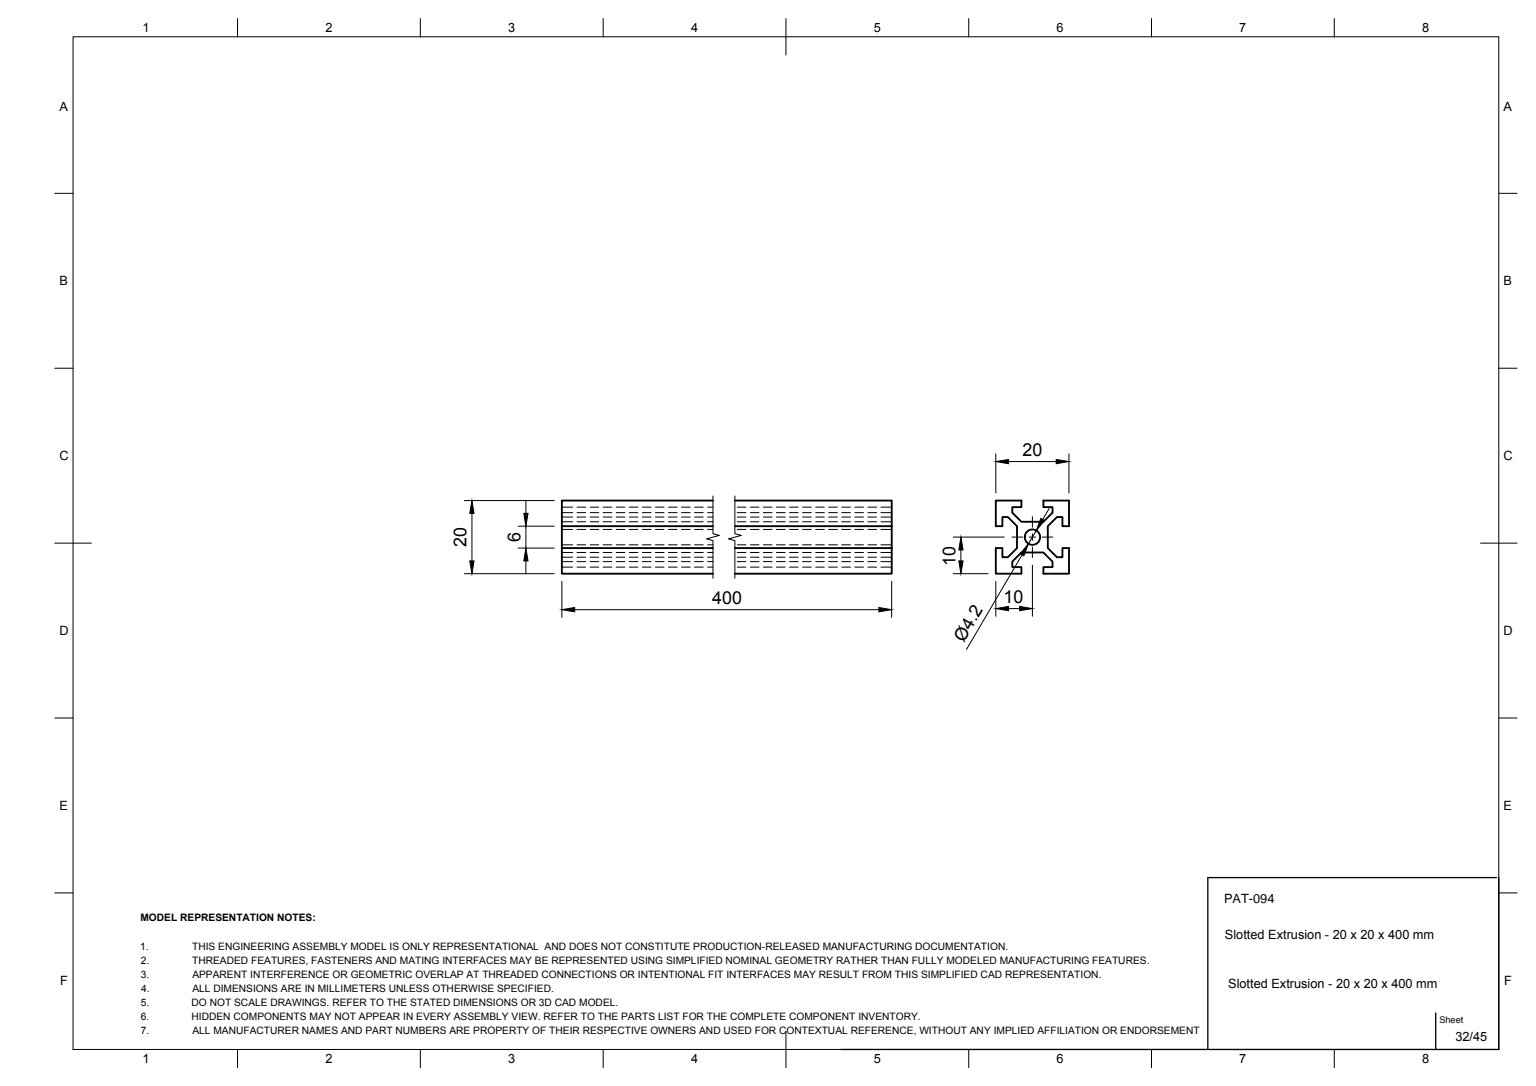
ISO-10303-21;
HEADER;
/* Generated by software containing ST-Developer
 * from STEP Tools, Inc. (www.steptools.com) 
 */

FILE_DESCRIPTION(
/* description */ ('Shaft runout checking stand'),
/* implementation_level */ '2;1');

FILE_NAME(
/* name */ 'Slotted Extrusion - 20 x 20 x 400 mm.step',
/* time_stamp */ '2026-11-02T21:12:33-08:00',
/* author */ (''),
/* organization */ (''),
/* preprocessor_version */ 'ST-DEVELOPER v20.2',
/* originating_system */ 'Autodesk Translation Framework v15.17.0.0',
/* authorisation */ '');

FILE_SCHEMA (('AUTOMOTIVE_DESIGN { 1 0 10303 214 3 1 1 }'));
ENDSEC;

DATA;
#10=MECHANICAL_DESIGN_GEOMETRIC_PRESENTATION_REPRESENTATION('',(#463),#11748);
#377=SHAPE_REPRESENTATION_RELATIONSHIP('SRR','None',#11926,#420);
#420=ADVANCED_BREP_SHAPE_REPRESENTATION('',(#514),#11702);
#463=STYLED_ITEM('',(#12169),#514);
#514=MANIFOLD_SOLID_BREP('Body1',#6206);
#562=FACE_BOUND('',#1452,.T.);
#563=FACE_BOUND('',#1454,.T.);
#673=CIRCLE('',#6774,0.21);
#674=CIRCLE('',#6775,0.21);
#938=CYLINDRICAL_SURFACE('',#6773,0.21);
#1038=FACE_OUTER_BOUND('',#1406,.T.);
#1039=FACE_OUTER_BOUND('',#1407,.T.);
#1040=FACE_OUTER_BOUND('',#1408,.T.);
#1041=FACE_OUTER_BOUND('',#1409,.T.);
#1042=FACE_OUTER_BOUND('',#1410,.T.);
#1043=FACE_OUTER_BOUND('',#1411,.T.);
#1044=FACE_OUTER_BOUND('',#1412,.T.);
#1045=FACE_OUTER_BOUND('',#1413,.T.);
#1046=FACE_OUTER_BOUND('',#1414,.T.);
#1047=FACE_OUTER_BOUND('',#1415,.T.);
#1048=FACE_OUTER_BOUND('',#1416,.T.);
#1049=FACE_OUTER_BOUND('',#1417,.T.);
#1050=FACE_OUTER_BOUND('',#1418,.T.);
#1051=FACE_OUTER_BOUND('',#1419,.T.);
#1052=FACE_OUTER_BOUND('',#1420,.T.);
#1053=FACE_OUTER_BOUND('',#1421,.T.);
#1054=FACE_OUTER_BOUND('',#1422,.T.);
#1055=FACE_OUTER_BOUND('',#1423,.T.);
#1056=FACE_OUTER_BOUND('',#1424,.T.);
#1057=FACE_OUTER_BOUND('',#1425,.T.);
#1058=FACE_OUTER_BOUND('',#1426,.T.);
#1059=FACE_OUTER_BOUND('',#1427,.T.);
#1060=FACE_OUTER_BOUND('',#1428,.T.);
#1061=FACE_OUTER_BOUND('',#1429,.T.);
#1062=FACE_OUTER_BOUND('',#1430,.T.);
#1063=FACE_OUTER_BOUND('',#1431,.T.);
#1064=FACE_OUTER_BOUND('',#1432,.T.);
#1065=FACE_OUTER_BOUND('',#1433,.T.);
#1066=FACE_OUTER_BOUND('',#1434,.T.);
#1067=FACE_OUTER_BOUND('',#1435,.T.);
#1068=FACE_OUTER_BOUND('',#1436,.T.);
#1069=FACE_OUTER_BOUND('',#1437,.T.);
#1070=FACE_OUTER_BOUND('',#1438,.T.);
#1071=FACE_OUTER_BOUND('',#1439,.T.);
#1072=FACE_OUTER_BOUND('',#1440,.T.);
#1073=FACE_OUTER_BOUND('',#1441,.T.);
#1074=FACE_OUTER_BOUND('',#1442,.T.);
#1075=FACE_OUTER_BOUND('',#1443,.T.);
#1076=FACE_OUTER_BOUND('',#1444,.T.);
#1077=FACE_OUTER_BOUND('',#1445,.T.);
#1078=FACE_OUTER_BOUND('',#1446,.T.);
#1079=FACE_OUTER_BOUND('',#1447,.T.);
#1080=FACE_OUTER_BOUND('',#1448,.T.);
#1081=FACE_OUTER_BOUND('',#1449,.T.);
#1082=FACE_OUTER_BOUND('',#1450,.T.);
#1083=FACE_OUTER_BOUND('',#1451,.T.);
#1084=FACE_OUTER_BOUND('',#1453,.T.);
#1406=EDGE_LOOP('',(#4088,#4089,#4090,#4091));
#1407=EDGE_LOOP('',(#4092,#4093,#4094,#4095));
#1408=EDGE_LOOP('',(#4096,#4097,#4098,#4099));
#1409=EDGE_LOOP('',(#4100,#4101,#4102,#4103));
#1410=EDGE_LOOP('',(#4104,#4105,#4106,#4107));
#1411=EDGE_LOOP('',(#4108,#4109,#4110,#4111));
#1412=EDGE_LOOP('',(#4112,#4113,#4114,#4115));
#1413=EDGE_LOOP('',(#4116,#4117,#4118,#4119));
#1414=EDGE_LOOP('',(#4120,#4121,#4122,#4123));
#1415=EDGE_LOOP('',(#4124,#4125,#4126,#4127));
#1416=EDGE_LOOP('',(#4128,#4129,#4130,#4131));
#1417=EDGE_LOOP('',(#4132,#4133,#4134,#4135));
#1418=EDGE_LOOP('',(#4136,#4137,#4138,#4139));
#1419=EDGE_LOOP('',(#4140,#4141,#4142,#4143));
#1420=EDGE_LOOP('',(#4144,#4145,#4146,#4147));
#1421=EDGE_LOOP('',(#4148,#4149,#4150,#4151));
#1422=EDGE_LOOP('',(#4152,#4153,#4154,#4155));
#1423=EDGE_LOOP('',(#4156,#4157,#4158,#4159));
#1424=EDGE_LOOP('',(#4160,#4161,#4162,#4163));
#1425=EDGE_LOOP('',(#4164,#4165,#4166,#4167));
#1426=EDGE_LOOP('',(#4168,#4169,#4170,#4171));
#1427=EDGE_LOOP('',(#4172,#4173,#4174,#4175));
#1428=EDGE_LOOP('',(#4176,#4177,#4178,#4179));
#1429=EDGE_LOOP('',(#4180,#4181,#4182,#4183));
#1430=EDGE_LOOP('',(#4184,#4185,#4186,#4187));
#1431=EDGE_LOOP('',(#4188,#4189,#4190,#4191));
#1432=EDGE_LOOP('',(#4192,#4193,#4194,#4195));
#1433=EDGE_LOOP('',(#4196,#4197,#4198,#4199));
#1434=EDGE_LOOP('',(#4200,#4201,#4202,#4203));
#1435=EDGE_LOOP('',(#4204,#4205,#4206,#4207));
#1436=EDGE_LOOP('',(#4208,#4209,#4210,#4211));
#1437=EDGE_LOOP('',(#4212,#4213,#4214,#4215));
#1438=EDGE_LOOP('',(#4216,#4217,#4218,#4219));
#1439=EDGE_LOOP('',(#4220,#4221,#4222,#4223));
#1440=EDGE_LOOP('',(#4224,#4225,#4226,#4227));
#1441=EDGE_LOOP('',(#4228,#4229,#4230,#4231));
#1442=EDGE_LOOP('',(#4232,#4233,#4234,#4235));
#1443=EDGE_LOOP('',(#4236,#4237,#4238,#4239));
#1444=EDGE_LOOP('',(#4240,#4241,#4242,#4243));
#1445=EDGE_LOOP('',(#4244,#4245,#4246,#4247));
#1446=EDGE_LOOP('',(#4248,#4249,#4250,#4251));
#1447=EDGE_LOOP('',(#4252,#4253,#4254,#4255));
#1448=EDGE_LOOP('',(#4256,#4257,#4258,#4259));
#1449=EDGE_LOOP('',(#4260,#4261,#4262,#4263));
#1450=EDGE_LOOP('',(#4264,#4265,#4266,#4267));
#1451=EDGE_LOOP('',(#4268,#4269,#4270,#4271,#4272,#4273,#4274,#4275,#4276,
#4277,#4278,#4279,#4280,#4281,#4282,#4283,#4284,#4285,#4286,#4287,#4288,
#4289,#4290,#4291,#4292,#4293,#4294,#4295,#4296,#4297,#4298,#4299,#4300,
#4301,#4302,#4303,#4304,#4305,#4306,#4307,#4308,#4309,#4310,#4311));
#1452=EDGE_LOOP('',(#4312));
#1453=EDGE_LOOP('',(#4313,#4314,#4315,#4316,#4317,#4318,#4319,#4320,#4321,
#4322,#4323,#4324,#4325,#4326,#4327,#4328,#4329,#4330,#4331,#4332,#4333,
#4334,#4335,#4336,#4337,#4338,#4339,#4340,#4341,#4342,#4343,#4344,#4345,
#4346,#4347,#4348,#4349,#4350,#4351,#4352,#4353,#4354,#4355,#4356));
#1454=EDGE_LOOP('',(#4357));
#1885=LINE('',#9481,#2352);
#1886=LINE('',#9483,#2353);
#1887=LINE('',#9485,#2354);
#1888=LINE('',#9486,#2355);
#1889=LINE('',#9489,#2356);
#1890=LINE('',#9491,#2357);
#1891=LINE('',#9492,#2358);
#1892=LINE('',#9495,#2359);
#1893=LINE('',#9497,#2360);
#1894=LINE('',#9498,#2361);
#1895=LINE('',#9501,#2362);
#1896=LINE('',#9503,#2363);
#1897=LINE('',#9504,#2364);
#1898=LINE('',#9507,#2365);
#1899=LINE('',#9509,#2366);
#1900=LINE('',#9510,#2367);
#1901=LINE('',#9513,#2368);
#1902=LINE('',#9515,#2369);
#1903=LINE('',#9516,#2370);
#1904=LINE('',#9519,#2371);
#1905=LINE('',#9521,#2372);
#1906=LINE('',#9522,#2373);
#1907=LINE('',#9525,#2374);
#1908=LINE('',#9527,#2375);
#1909=LINE('',#9528,#2376);
#1910=LINE('',#9531,#2377);
#1911=LINE('',#9533,#2378);
#1912=LINE('',#9534,#2379);
#1913=LINE('',#9538,#2380);
#1914=LINE('',#9540,#2381);
#1915=LINE('',#9542,#2382);
#1916=LINE('',#9543,#2383);
#1917=LINE('',#9546,#2384);
#1918=LINE('',#9548,#2385);
#1919=LINE('',#9549,#2386);
#1920=LINE('',#9552,#2387);
#1921=LINE('',#9554,#2388);
#1922=LINE('',#9555,#2389);
#1923=LINE('',#9558,#2390);
#1924=LINE('',#9560,#2391);
#1925=LINE('',#9561,#2392);
#1926=LINE('',#9564,#2393);
#1927=LINE('',#9566,#2394);
#1928=LINE('',#9567,#2395);
#1929=LINE('',#9570,#2396);
#1930=LINE('',#9572,#2397);
#1931=LINE('',#9573,#2398);
#1932=LINE('',#9576,#2399);
#1933=LINE('',#9578,#2400);
#1934=LINE('',#9579,#2401);
#1935=LINE('',#9582,#2402);
#1936=LINE('',#9584,#2403);
#1937=LINE('',#9585,#2404);
#1938=LINE('',#9588,#2405);
#1939=LINE('',#9590,#2406);
#1940=LINE('',#9591,#2407);
#1941=LINE('',#9595,#2408);
#1942=LINE('',#9597,#2409);
#1943=LINE('',#9599,#2410);
#1944=LINE('',#9600,#2411);
#1945=LINE('',#9603,#2412);
#1946=LINE('',#9605,#2413);
#1947=LINE('',#9606,#2414);
#1948=LINE('',#9609,#2415);
#1949=LINE('',#9611,#2416);
#1950=LINE('',#9612,#2417);
#1951=LINE('',#9615,#2418);
#1952=LINE('',#9617,#2419);
#1953=LINE('',#9618,#2420);
#1954=LINE('',#9621,#2421);
#1955=LINE('',#9623,#2422);
#1956=LINE('',#9624,#2423);
#1957=LINE('',#9627,#2424);
#1958=LINE('',#9629,#2425);
#1959=LINE('',#9630,#2426);
#1960=LINE('',#9633,#2427);
#1961=LINE('',#9635,#2428);
#1962=LINE('',#9636,#2429);
#1963=LINE('',#9639,#2430);
#1964=LINE('',#9641,#2431);
#1965=LINE('',#9642,#2432);
#1966=LINE('',#9645,#2433);
#1967=LINE('',#9647,#2434);
#1968=LINE('',#9648,#2435);
#1969=LINE('',#9652,#2436);
#1970=LINE('',#9654,#2437);
#1971=LINE('',#9656,#2438);
#1972=LINE('',#9657,#2439);
#1973=LINE('',#9660,#2440);
#1974=LINE('',#9662,#2441);
#1975=LINE('',#9663,#2442);
#1976=LINE('',#9666,#2443);
#1977=LINE('',#9668,#2444);
#1978=LINE('',#9669,#2445);
#1979=LINE('',#9672,#2446);
#1980=LINE('',#9674,#2447);
#1981=LINE('',#9675,#2448);
#1982=LINE('',#9678,#2449);
#1983=LINE('',#9680,#2450);
#1984=LINE('',#9681,#2451);
#1985=LINE('',#9684,#2452);
#1986=LINE('',#9686,#2453);
#1987=LINE('',#9687,#2454);
#1988=LINE('',#9690,#2455);
#1989=LINE('',#9692,#2456);
#1990=LINE('',#9693,#2457);
#1991=LINE('',#9696,#2458);
#1992=LINE('',#9698,#2459);
#1993=LINE('',#9699,#2460);
#1994=LINE('',#9702,#2461);
#1995=LINE('',#9704,#2462);
#1996=LINE('',#9705,#2463);
#1997=LINE('',#9710,#2464);
#1998=LINE('',#9714,#2465);
#1999=LINE('',#9716,#2466);
#2000=LINE('',#9717,#2467);
#2001=LINE('',#9720,#2468);
#2002=LINE('',#9722,#2469);
#2003=LINE('',#9723,#2470);
#2004=LINE('',#9725,#2471);
#2005=LINE('',#9726,#2472);
#2006=LINE('',#9729,#2473);
#2007=LINE('',#9731,#2474);
#2008=LINE('',#9732,#2475);
#2009=LINE('',#9734,#2476);
#2010=LINE('',#9735,#2477);
#2011=LINE('',#9738,#2478);
#2012=LINE('',#9740,#2479);
#2013=LINE('',#9741,#2480);
#2014=LINE('',#9743,#2481);
#2015=LINE('',#9744,#2482);
#2016=LINE('',#9746,#2483);
#2017=LINE('',#9747,#2484);
#2352=VECTOR('',#7500,1.);
#2353=VECTOR('',#7501,1.);
#2354=VECTOR('',#7502,1.);
#2355=VECTOR('',#7503,1.);
#2356=VECTOR('',#7506,1.);
#2357=VECTOR('',#7507,1.);
#2358=VECTOR('',#7508,1.);
#2359=VECTOR('',#7511,1.);
#2360=VECTOR('',#7512,1.);
#2361=VECTOR('',#7513,1.);
#2362=VECTOR('',#7516,1.);
#2363=VECTOR('',#7517,1.);
#2364=VECTOR('',#7518,1.);
#2365=VECTOR('',#7521,1.);
#2366=VECTOR('',#7522,1.);
#2367=VECTOR('',#7523,1.);
#2368=VECTOR('',#7526,1.);
#2369=VECTOR('',#7527,1.);
#2370=VECTOR('',#7528,1.);
#2371=VECTOR('',#7531,1.);
#2372=VECTOR('',#7532,1.);
#2373=VECTOR('',#7533,1.);
#2374=VECTOR('',#7536,1.);
#2375=VECTOR('',#7537,1.);
#2376=VECTOR('',#7538,1.);
#2377=VECTOR('',#7541,1.);
#2378=VECTOR('',#7542,1.);
#2379=VECTOR('',#7543,1.);
#2380=VECTOR('',#7546,1.);
#2381=VECTOR('',#7547,1.);
#2382=VECTOR('',#7548,1.);
#2383=VECTOR('',#7549,1.);
#2384=VECTOR('',#7552,1.);
#2385=VECTOR('',#7553,1.);
#2386=VECTOR('',#7554,1.);
#2387=VECTOR('',#7557,1.);
#2388=VECTOR('',#7558,1.);
#2389=VECTOR('',#7559,1.);
#2390=VECTOR('',#7562,1.);
#2391=VECTOR('',#7563,1.);
#2392=VECTOR('',#7564,1.);
#2393=VECTOR('',#7567,1.);
#2394=VECTOR('',#7568,1.);
#2395=VECTOR('',#7569,1.);
#2396=VECTOR('',#7572,1.);
#2397=VECTOR('',#7573,1.);
#2398=VECTOR('',#7574,1.);
#2399=VECTOR('',#7577,1.);
#2400=VECTOR('',#7578,1.);
#2401=VECTOR('',#7579,1.);
#2402=VECTOR('',#7582,1.);
#2403=VECTOR('',#7583,1.);
#2404=VECTOR('',#7584,1.);
#2405=VECTOR('',#7587,1.);
#2406=VECTOR('',#7588,1.);
#2407=VECTOR('',#7589,1.);
#2408=VECTOR('',#7592,1.);
#2409=VECTOR('',#7593,1.);
#2410=VECTOR('',#7594,1.);
#2411=VECTOR('',#7595,1.);
#2412=VECTOR('',#7598,1.);
#2413=VECTOR('',#7599,1.);
#2414=VECTOR('',#7600,1.);
#2415=VECTOR('',#7603,1.);
#2416=VECTOR('',#7604,1.);
#2417=VECTOR('',#7605,1.);
#2418=VECTOR('',#7608,1.);
#2419=VECTOR('',#7609,1.);
#2420=VECTOR('',#7610,1.);
#2421=VECTOR('',#7613,1.);
#2422=VECTOR('',#7614,1.);
#2423=VECTOR('',#7615,1.);
#2424=VECTOR('',#7618,1.);
#2425=VECTOR('',#7619,1.);
#2426=VECTOR('',#7620,1.);
#2427=VECTOR('',#7623,1.);
#2428=VECTOR('',#7624,1.);
#2429=VECTOR('',#7625,1.);
#2430=VECTOR('',#7628,1.);
#2431=VECTOR('',#7629,1.);
#2432=VECTOR('',#7630,1.);
#2433=VECTOR('',#7633,1.);
#2434=VECTOR('',#7634,1.);
#2435=VECTOR('',#7635,1.);
#2436=VECTOR('',#7638,1.);
#2437=VECTOR('',#7639,1.);
#2438=VECTOR('',#7640,1.);
#2439=VECTOR('',#7641,1.);
#2440=VECTOR('',#7644,1.);
#2441=VECTOR('',#7645,1.);
#2442=VECTOR('',#7646,1.);
#2443=VECTOR('',#7649,1.);
#2444=VECTOR('',#7650,1.);
#2445=VECTOR('',#7651,1.);
#2446=VECTOR('',#7654,1.);
#2447=VECTOR('',#7655,1.);
#2448=VECTOR('',#7656,1.);
#2449=VECTOR('',#7659,1.);
#2450=VECTOR('',#7660,1.);
#2451=VECTOR('',#7661,1.);
#2452=VECTOR('',#7664,1.);
#2453=VECTOR('',#7665,1.);
#2454=VECTOR('',#7666,1.);
#2455=VECTOR('',#7669,1.);
#2456=VECTOR('',#7670,1.);
#2457=VECTOR('',#7671,1.);
#2458=VECTOR('',#7674,1.);
#2459=VECTOR('',#7675,1.);
#2460=VECTOR('',#7676,1.);
#2461=VECTOR('',#7679,1.);
#2462=VECTOR('',#7680,1.);
#2463=VECTOR('',#7681,1.);
#2464=VECTOR('',#7686,0.21);
#2465=VECTOR('',#7691,1.);
#2466=VECTOR('',#7692,1.);
#2467=VECTOR('',#7693,1.);
#2468=VECTOR('',#7696,1.);
#2469=VECTOR('',#7697,1.);
#2470=VECTOR('',#7698,1.);
#2471=VECTOR('',#7701,1.);
#2472=VECTOR('',#7702,1.);
#2473=VECTOR('',#7705,1.);
#2474=VECTOR('',#7706,1.);
#2475=VECTOR('',#7707,1.);
#2476=VECTOR('',#7710,1.);
#2477=VECTOR('',#7711,1.);
#2478=VECTOR('',#7714,1.);
#2479=VECTOR('',#7715,1.);
#2480=VECTOR('',#7716,1.);
#2481=VECTOR('',#7719,1.);
#2482=VECTOR('',#7720,1.);
#2483=VECTOR('',#7723,1.);
#2484=VECTOR('',#7724,1.);
#2819=VERTEX_POINT('',#9479);
#2820=VERTEX_POINT('',#9480);
#2821=VERTEX_POINT('',#9482);
#2822=VERTEX_POINT('',#9484);
#2823=VERTEX_POINT('',#9488);
#2824=VERTEX_POINT('',#9490);
#2825=VERTEX_POINT('',#9494);
#2826=VERTEX_POINT('',#9496);
#2827=VERTEX_POINT('',#9500);
#2828=VERTEX_POINT('',#9502);
#2829=VERTEX_POINT('',#9506);
#2830=VERTEX_POINT('',#9508);
#2831=VERTEX_POINT('',#9512);
#2832=VERTEX_POINT('',#9514);
#2833=VERTEX_POINT('',#9518);
#2834=VERTEX_POINT('',#9520);
#2835=VERTEX_POINT('',#9524);
#2836=VERTEX_POINT('',#9526);
#2837=VERTEX_POINT('',#9530);
#2838=VERTEX_POINT('',#9532);
#2839=VERTEX_POINT('',#9536);
#2840=VERTEX_POINT('',#9537);
#2841=VERTEX_POINT('',#9539);
#2842=VERTEX_POINT('',#9541);
#2843=VERTEX_POINT('',#9545);
#2844=VERTEX_POINT('',#9547);
#2845=VERTEX_POINT('',#9551);
#2846=VERTEX_POINT('',#9553);
#2847=VERTEX_POINT('',#9557);
#2848=VERTEX_POINT('',#9559);
#2849=VERTEX_POINT('',#9563);
#2850=VERTEX_POINT('',#9565);
#2851=VERTEX_POINT('',#9569);
#2852=VERTEX_POINT('',#9571);
#2853=VERTEX_POINT('',#9575);
#2854=VERTEX_POINT('',#9577);
#2855=VERTEX_POINT('',#9581);
#2856=VERTEX_POINT('',#9583);
#2857=VERTEX_POINT('',#9587);
#2858=VERTEX_POINT('',#9589);
#2859=VERTEX_POINT('',#9593);
#2860=VERTEX_POINT('',#9594);
#2861=VERTEX_POINT('',#9596);
#2862=VERTEX_POINT('',#9598);
#2863=VERTEX_POINT('',#9602);
#2864=VERTEX_POINT('',#9604);
#2865=VERTEX_POINT('',#9608);
#2866=VERTEX_POINT('',#9610);
#2867=VERTEX_POINT('',#9614);
#2868=VERTEX_POINT('',#9616);
#2869=VERTEX_POINT('',#9620);
#2870=VERTEX_POINT('',#9622);
#2871=VERTEX_POINT('',#9626);
#2872=VERTEX_POINT('',#9628);
#2873=VERTEX_POINT('',#9632);
#2874=VERTEX_POINT('',#9634);
#2875=VERTEX_POINT('',#9638);
#2876=VERTEX_POINT('',#9640);
#2877=VERTEX_POINT('',#9644);
#2878=VERTEX_POINT('',#9646);
#2879=VERTEX_POINT('',#9650);
#2880=VERTEX_POINT('',#9651);
#2881=VERTEX_POINT('',#9653);
#2882=VERTEX_POINT('',#9655);
#2883=VERTEX_POINT('',#9659);
#2884=VERTEX_POINT('',#9661);
#2885=VERTEX_POINT('',#9665);
#2886=VERTEX_POINT('',#9667);
#2887=VERTEX_POINT('',#9671);
#2888=VERTEX_POINT('',#9673);
#2889=VERTEX_POINT('',#9677);
#2890=VERTEX_POINT('',#9679);
#2891=VERTEX_POINT('',#9683);
#2892=VERTEX_POINT('',#9685);
#2893=VERTEX_POINT('',#9689);
#2894=VERTEX_POINT('',#9691);
#2895=VERTEX_POINT('',#9695);
#2896=VERTEX_POINT('',#9697);
#2897=VERTEX_POINT('',#9701);
#2898=VERTEX_POINT('',#9703);
#2899=VERTEX_POINT('',#9707);
#2900=VERTEX_POINT('',#9709);
#2901=VERTEX_POINT('',#9713);
#2902=VERTEX_POINT('',#9715);
#2903=VERTEX_POINT('',#9719);
#2904=VERTEX_POINT('',#9721);
#2905=VERTEX_POINT('',#9728);
#2906=VERTEX_POINT('',#9730);
#2907=VERTEX_POINT('',#9737);
#2908=VERTEX_POINT('',#9739);
#3330=EDGE_CURVE('',#2819,#2820,#1885,.T.);
#3331=EDGE_CURVE('',#2819,#2821,#1886,.T.);
#3332=EDGE_CURVE('',#2822,#2821,#1887,.T.);
#3333=EDGE_CURVE('',#2820,#2822,#1888,.T.);
#3334=EDGE_CURVE('',#2823,#2819,#1889,.T.);
#3335=EDGE_CURVE('',#2823,#2824,#1890,.T.);
#3336=EDGE_CURVE('',#2821,#2824,#1891,.T.);
#3337=EDGE_CURVE('',#2825,#2823,#1892,.T.);
#3338=EDGE_CURVE('',#2825,#2826,#1893,.T.);
#3339=EDGE_CURVE('',#2824,#2826,#1894,.T.);
#3340=EDGE_CURVE('',#2827,#2825,#1895,.T.);
#3341=EDGE_CURVE('',#2827,#2828,#1896,.T.);
#3342=EDGE_CURVE('',#2826,#2828,#1897,.T.);
#3343=EDGE_CURVE('',#2829,#2827,#1898,.T.);
#3344=EDGE_CURVE('',#2829,#2830,#1899,.T.);
#3345=EDGE_CURVE('',#2828,#2830,#1900,.T.);
#3346=EDGE_CURVE('',#2831,#2829,#1901,.T.);
#3347=EDGE_CURVE('',#2831,#2832,#1902,.T.);
#3348=EDGE_CURVE('',#2830,#2832,#1903,.T.);
#3349=EDGE_CURVE('',#2833,#2831,#1904,.T.);
#3350=EDGE_CURVE('',#2833,#2834,#1905,.T.);
#3351=EDGE_CURVE('',#2832,#2834,#1906,.T.);
#3352=EDGE_CURVE('',#2835,#2833,#1907,.T.);
#3353=EDGE_CURVE('',#2835,#2836,#1908,.T.);
#3354=EDGE_CURVE('',#2834,#2836,#1909,.T.);
#3355=EDGE_CURVE('',#2837,#2835,#1910,.T.);
#3356=EDGE_CURVE('',#2838,#2837,#1911,.T.);
#3357=EDGE_CURVE('',#2836,#2838,#1912,.T.);
#3358=EDGE_CURVE('',#2839,#2840,#1913,.T.);
#3359=EDGE_CURVE('',#2839,#2841,#1914,.T.);
#3360=EDGE_CURVE('',#2842,#2841,#1915,.T.);
#3361=EDGE_CURVE('',#2840,#2842,#1916,.T.);
#3362=EDGE_CURVE('',#2843,#2839,#1917,.T.);
#3363=EDGE_CURVE('',#2843,#2844,#1918,.T.);
#3364=EDGE_CURVE('',#2841,#2844,#1919,.T.);
#3365=EDGE_CURVE('',#2845,#2843,#1920,.T.);
#3366=EDGE_CURVE('',#2845,#2846,#1921,.T.);
#3367=EDGE_CURVE('',#2844,#2846,#1922,.T.);
#3368=EDGE_CURVE('',#2847,#2845,#1923,.T.);
#3369=EDGE_CURVE('',#2847,#2848,#1924,.T.);
#3370=EDGE_CURVE('',#2846,#2848,#1925,.T.);
#3371=EDGE_CURVE('',#2849,#2847,#1926,.T.);
#3372=EDGE_CURVE('',#2849,#2850,#1927,.T.);
#3373=EDGE_CURVE('',#2848,#2850,#1928,.T.);
#3374=EDGE_CURVE('',#2851,#2849,#1929,.T.);
#3375=EDGE_CURVE('',#2851,#2852,#1930,.T.);
#3376=EDGE_CURVE('',#2850,#2852,#1931,.T.);
#3377=EDGE_CURVE('',#2853,#2851,#1932,.T.);
#3378=EDGE_CURVE('',#2853,#2854,#1933,.T.);
#3379=EDGE_CURVE('',#2852,#2854,#1934,.T.);
#3380=EDGE_CURVE('',#2855,#2853,#1935,.T.);
#3381=EDGE_CURVE('',#2855,#2856,#1936,.T.);
#3382=EDGE_CURVE('',#2854,#2856,#1937,.T.);
#3383=EDGE_CURVE('',#2857,#2855,#1938,.T.);
#3384=EDGE_CURVE('',#2858,#2857,#1939,.T.);
#3385=EDGE_CURVE('',#2856,#2858,#1940,.T.);
#3386=EDGE_CURVE('',#2859,#2860,#1941,.T.);
#3387=EDGE_CURVE('',#2859,#2861,#1942,.T.);
#3388=EDGE_CURVE('',#2862,#2861,#1943,.T.);
#3389=EDGE_CURVE('',#2860,#2862,#1944,.T.);
#3390=EDGE_CURVE('',#2863,#2859,#1945,.T.);
#3391=EDGE_CURVE('',#2863,#2864,#1946,.T.);
#3392=EDGE_CURVE('',#2861,#2864,#1947,.T.);
#3393=EDGE_CURVE('',#2865,#2863,#1948,.T.);
#3394=EDGE_CURVE('',#2865,#2866,#1949,.T.);
#3395=EDGE_CURVE('',#2864,#2866,#1950,.T.);
#3396=EDGE_CURVE('',#2867,#2865,#1951,.T.);
#3397=EDGE_CURVE('',#2867,#2868,#1952,.T.);
#3398=EDGE_CURVE('',#2866,#2868,#1953,.T.);
#3399=EDGE_CURVE('',#2869,#2867,#1954,.T.);
#3400=EDGE_CURVE('',#2869,#2870,#1955,.T.);
#3401=EDGE_CURVE('',#2868,#2870,#1956,.T.);
#3402=EDGE_CURVE('',#2871,#2869,#1957,.T.);
#3403=EDGE_CURVE('',#2871,#2872,#1958,.T.);
#3404=EDGE_CURVE('',#2870,#2872,#1959,.T.);
#3405=EDGE_CURVE('',#2873,#2871,#1960,.T.);
#3406=EDGE_CURVE('',#2873,#2874,#1961,.T.);
#3407=EDGE_CURVE('',#2872,#2874,#1962,.T.);
#3408=EDGE_CURVE('',#2875,#2873,#1963,.T.);
#3409=EDGE_CURVE('',#2875,#2876,#1964,.T.);
#3410=EDGE_CURVE('',#2874,#2876,#1965,.T.);
#3411=EDGE_CURVE('',#2877,#2875,#1966,.T.);
#3412=EDGE_CURVE('',#2878,#2877,#1967,.T.);
#3413=EDGE_CURVE('',#2876,#2878,#1968,.T.);
#3414=EDGE_CURVE('',#2879,#2880,#1969,.T.);
#3415=EDGE_CURVE('',#2879,#2881,#1970,.T.);
#3416=EDGE_CURVE('',#2882,#2881,#1971,.T.);
#3417=EDGE_CURVE('',#2880,#2882,#1972,.T.);
#3418=EDGE_CURVE('',#2883,#2879,#1973,.T.);
#3419=EDGE_CURVE('',#2883,#2884,#1974,.T.);
#3420=EDGE_CURVE('',#2881,#2884,#1975,.T.);
#3421=EDGE_CURVE('',#2885,#2883,#1976,.T.);
#3422=EDGE_CURVE('',#2885,#2886,#1977,.T.);
#3423=EDGE_CURVE('',#2884,#2886,#1978,.T.);
#3424=EDGE_CURVE('',#2887,#2885,#1979,.T.);
#3425=EDGE_CURVE('',#2887,#2888,#1980,.T.);
#3426=EDGE_CURVE('',#2886,#2888,#1981,.T.);
#3427=EDGE_CURVE('',#2889,#2887,#1982,.T.);
#3428=EDGE_CURVE('',#2889,#2890,#1983,.T.);
#3429=EDGE_CURVE('',#2888,#2890,#1984,.T.);
#3430=EDGE_CURVE('',#2891,#2889,#1985,.T.);
#3431=EDGE_CURVE('',#2891,#2892,#1986,.T.);
#3432=EDGE_CURVE('',#2890,#2892,#1987,.T.);
#3433=EDGE_CURVE('',#2893,#2891,#1988,.T.);
#3434=EDGE_CURVE('',#2893,#2894,#1989,.T.);
#3435=EDGE_CURVE('',#2892,#2894,#1990,.T.);
#3436=EDGE_CURVE('',#2895,#2893,#1991,.T.);
#3437=EDGE_CURVE('',#2895,#2896,#1992,.T.);
#3438=EDGE_CURVE('',#2894,#2896,#1993,.T.);
#3439=EDGE_CURVE('',#2897,#2895,#1994,.T.);
#3440=EDGE_CURVE('',#2898,#2897,#1995,.T.);
#3441=EDGE_CURVE('',#2896,#2898,#1996,.T.);
#3442=EDGE_CURVE('',#2899,#2899,#673,.T.);
#3443=EDGE_CURVE('',#2899,#2900,#1997,.T.);
#3444=EDGE_CURVE('',#2900,#2900,#674,.T.);
#3445=EDGE_CURVE('',#2837,#2901,#1998,.T.);
#3446=EDGE_CURVE('',#2901,#2902,#1999,.T.);
#3447=EDGE_CURVE('',#2838,#2902,#2000,.T.);
#3448=EDGE_CURVE('',#2903,#2822,#2001,.T.);
#3449=EDGE_CURVE('',#2904,#2903,#2002,.T.);
#3450=EDGE_CURVE('',#2904,#2820,#2003,.T.);
#3451=EDGE_CURVE('',#2857,#2904,#2004,.T.);
#3452=EDGE_CURVE('',#2858,#2903,#2005,.T.);
#3453=EDGE_CURVE('',#2905,#2842,#2006,.T.);
#3454=EDGE_CURVE('',#2906,#2905,#2007,.T.);
#3455=EDGE_CURVE('',#2906,#2840,#2008,.T.);
#3456=EDGE_CURVE('',#2877,#2906,#2009,.T.);
#3457=EDGE_CURVE('',#2878,#2905,#2010,.T.);
#3458=EDGE_CURVE('',#2907,#2862,#2011,.T.);
#3459=EDGE_CURVE('',#2908,#2907,#2012,.T.);
#3460=EDGE_CURVE('',#2908,#2860,#2013,.T.);
#3461=EDGE_CURVE('',#2897,#2908,#2014,.T.);
#3462=EDGE_CURVE('',#2898,#2907,#2015,.T.);
#3463=EDGE_CURVE('',#2902,#2882,#2016,.T.);
#3464=EDGE_CURVE('',#2901,#2880,#2017,.T.);
#4088=ORIENTED_EDGE('',*,*,#3330,.F.);
#4089=ORIENTED_EDGE('',*,*,#3331,.T.);
#4090=ORIENTED_EDGE('',*,*,#3332,.F.);
#4091=ORIENTED_EDGE('',*,*,#3333,.F.);
#4092=ORIENTED_EDGE('',*,*,#3334,.F.);
#4093=ORIENTED_EDGE('',*,*,#3335,.T.);
#4094=ORIENTED_EDGE('',*,*,#3336,.F.);
#4095=ORIENTED_EDGE('',*,*,#3331,.F.);
#4096=ORIENTED_EDGE('',*,*,#3337,.F.);
#4097=ORIENTED_EDGE('',*,*,#3338,.T.);
#4098=ORIENTED_EDGE('',*,*,#3339,.F.);
#4099=ORIENTED_EDGE('',*,*,#3335,.F.);
#4100=ORIENTED_EDGE('',*,*,#3340,.F.);
#4101=ORIENTED_EDGE('',*,*,#3341,.T.);
#4102=ORIENTED_EDGE('',*,*,#3342,.F.);
#4103=ORIENTED_EDGE('',*,*,#3338,.F.);
#4104=ORIENTED_EDGE('',*,*,#3343,.F.);
#4105=ORIENTED_EDGE('',*,*,#3344,.T.);
#4106=ORIENTED_EDGE('',*,*,#3345,.F.);
#4107=ORIENTED_EDGE('',*,*,#3341,.F.);
#4108=ORIENTED_EDGE('',*,*,#3346,.F.);
#4109=ORIENTED_EDGE('',*,*,#3347,.T.);
#4110=ORIENTED_EDGE('',*,*,#3348,.F.);
#4111=ORIENTED_EDGE('',*,*,#3344,.F.);
#4112=ORIENTED_EDGE('',*,*,#3349,.F.);
#4113=ORIENTED_EDGE('',*,*,#3350,.T.);
#4114=ORIENTED_EDGE('',*,*,#3351,.F.);
#4115=ORIENTED_EDGE('',*,*,#3347,.F.);
#4116=ORIENTED_EDGE('',*,*,#3352,.F.);
#4117=ORIENTED_EDGE('',*,*,#3353,.T.);
#4118=ORIENTED_EDGE('',*,*,#3354,.F.);
#4119=ORIENTED_EDGE('',*,*,#3350,.F.);
#4120=ORIENTED_EDGE('',*,*,#3355,.F.);
#4121=ORIENTED_EDGE('',*,*,#3356,.F.);
#4122=ORIENTED_EDGE('',*,*,#3357,.F.);
#4123=ORIENTED_EDGE('',*,*,#3353,.F.);
#4124=ORIENTED_EDGE('',*,*,#3358,.F.);
#4125=ORIENTED_EDGE('',*,*,#3359,.T.);
#4126=ORIENTED_EDGE('',*,*,#3360,.F.);
#4127=ORIENTED_EDGE('',*,*,#3361,.F.);
#4128=ORIENTED_EDGE('',*,*,#3362,.F.);
#4129=ORIENTED_EDGE('',*,*,#3363,.T.);
#4130=ORIENTED_EDGE('',*,*,#3364,.F.);
#4131=ORIENTED_EDGE('',*,*,#3359,.F.);
#4132=ORIENTED_EDGE('',*,*,#3365,.F.);
#4133=ORIENTED_EDGE('',*,*,#3366,.T.);
#4134=ORIENTED_EDGE('',*,*,#3367,.F.);
#4135=ORIENTED_EDGE('',*,*,#3363,.F.);
#4136=ORIENTED_EDGE('',*,*,#3368,.F.);
#4137=ORIENTED_EDGE('',*,*,#3369,.T.);
#4138=ORIENTED_EDGE('',*,*,#3370,.F.);
#4139=ORIENTED_EDGE('',*,*,#3366,.F.);
#4140=ORIENTED_EDGE('',*,*,#3371,.F.);
#4141=ORIENTED_EDGE('',*,*,#3372,.T.);
#4142=ORIENTED_EDGE('',*,*,#3373,.F.);
#4143=ORIENTED_EDGE('',*,*,#3369,.F.);
#4144=ORIENTED_EDGE('',*,*,#3374,.F.);
#4145=ORIENTED_EDGE('',*,*,#3375,.T.);
#4146=ORIENTED_EDGE('',*,*,#3376,.F.);
#4147=ORIENTED_EDGE('',*,*,#3372,.F.);
#4148=ORIENTED_EDGE('',*,*,#3377,.F.);
#4149=ORIENTED_EDGE('',*,*,#3378,.T.);
#4150=ORIENTED_EDGE('',*,*,#3379,.F.);
#4151=ORIENTED_EDGE('',*,*,#3375,.F.);
#4152=ORIENTED_EDGE('',*,*,#3380,.F.);
#4153=ORIENTED_EDGE('',*,*,#3381,.T.);
#4154=ORIENTED_EDGE('',*,*,#3382,.F.);
#4155=ORIENTED_EDGE('',*,*,#3378,.F.);
#4156=ORIENTED_EDGE('',*,*,#3383,.F.);
#4157=ORIENTED_EDGE('',*,*,#3384,.F.);
#4158=ORIENTED_EDGE('',*,*,#3385,.F.);
#4159=ORIENTED_EDGE('',*,*,#3381,.F.);
#4160=ORIENTED_EDGE('',*,*,#3386,.F.);
#4161=ORIENTED_EDGE('',*,*,#3387,.T.);
#4162=ORIENTED_EDGE('',*,*,#3388,.F.);
#4163=ORIENTED_EDGE('',*,*,#3389,.F.);
#4164=ORIENTED_EDGE('',*,*,#3390,.F.);
#4165=ORIENTED_EDGE('',*,*,#3391,.T.);
#4166=ORIENTED_EDGE('',*,*,#3392,.F.);
#4167=ORIENTED_EDGE('',*,*,#3387,.F.);
#4168=ORIENTED_EDGE('',*,*,#3393,.F.);
#4169=ORIENTED_EDGE('',*,*,#3394,.T.);
#4170=ORIENTED_EDGE('',*,*,#3395,.F.);
#4171=ORIENTED_EDGE('',*,*,#3391,.F.);
#4172=ORIENTED_EDGE('',*,*,#3396,.F.);
#4173=ORIENTED_EDGE('',*,*,#3397,.T.);
#4174=ORIENTED_EDGE('',*,*,#3398,.F.);
#4175=ORIENTED_EDGE('',*,*,#3394,.F.);
#4176=ORIENTED_EDGE('',*,*,#3399,.F.);
#4177=ORIENTED_EDGE('',*,*,#3400,.T.);
#4178=ORIENTED_EDGE('',*,*,#3401,.F.);
#4179=ORIENTED_EDGE('',*,*,#3397,.F.);
#4180=ORIENTED_EDGE('',*,*,#3402,.F.);
#4181=ORIENTED_EDGE('',*,*,#3403,.T.);
#4182=ORIENTED_EDGE('',*,*,#3404,.F.);
#4183=ORIENTED_EDGE('',*,*,#3400,.F.);
#4184=ORIENTED_EDGE('',*,*,#3405,.F.);
#4185=ORIENTED_EDGE('',*,*,#3406,.T.);
#4186=ORIENTED_EDGE('',*,*,#3407,.F.);
#4187=ORIENTED_EDGE('',*,*,#3403,.F.);
#4188=ORIENTED_EDGE('',*,*,#3408,.F.);
#4189=ORIENTED_EDGE('',*,*,#3409,.T.);
#4190=ORIENTED_EDGE('',*,*,#3410,.F.);
#4191=ORIENTED_EDGE('',*,*,#3406,.F.);
#4192=ORIENTED_EDGE('',*,*,#3411,.F.);
#4193=ORIENTED_EDGE('',*,*,#3412,.F.);
#4194=ORIENTED_EDGE('',*,*,#3413,.F.);
#4195=ORIENTED_EDGE('',*,*,#3409,.F.);
#4196=ORIENTED_EDGE('',*,*,#3414,.F.);
#4197=ORIENTED_EDGE('',*,*,#3415,.T.);
#4198=ORIENTED_EDGE('',*,*,#3416,.F.);
#4199=ORIENTED_EDGE('',*,*,#3417,.F.);
#4200=ORIENTED_EDGE('',*,*,#3418,.F.);
#4201=ORIENTED_EDGE('',*,*,#3419,.T.);
#4202=ORIENTED_EDGE('',*,*,#3420,.F.);
#4203=ORIENTED_EDGE('',*,*,#3415,.F.);
#4204=ORIENTED_EDGE('',*,*,#3421,.F.);
#4205=ORIENTED_EDGE('',*,*,#3422,.T.);
#4206=ORIENTED_EDGE('',*,*,#3423,.F.);
#4207=ORIENTED_EDGE('',*,*,#3419,.F.);
#4208=ORIENTED_EDGE('',*,*,#3424,.F.);
#4209=ORIENTED_EDGE('',*,*,#3425,.T.);
#4210=ORIENTED_EDGE('',*,*,#3426,.F.);
#4211=ORIENTED_EDGE('',*,*,#3422,.F.);
#4212=ORIENTED_EDGE('',*,*,#3427,.F.);
#4213=ORIENTED_EDGE('',*,*,#3428,.T.);
#4214=ORIENTED_EDGE('',*,*,#3429,.F.);
#4215=ORIENTED_EDGE('',*,*,#3425,.F.);
#4216=ORIENTED_EDGE('',*,*,#3430,.F.);
#4217=ORIENTED_EDGE('',*,*,#3431,.T.);
#4218=ORIENTED_EDGE('',*,*,#3432,.F.);
#4219=ORIENTED_EDGE('',*,*,#3428,.F.);
#4220=ORIENTED_EDGE('',*,*,#3433,.F.);
#4221=ORIENTED_EDGE('',*,*,#3434,.T.);
#4222=ORIENTED_EDGE('',*,*,#3435,.F.);
#4223=ORIENTED_EDGE('',*,*,#3431,.F.);
#4224=ORIENTED_EDGE('',*,*,#3436,.F.);
#4225=ORIENTED_EDGE('',*,*,#3437,.T.);
#4226=ORIENTED_EDGE('',*,*,#3438,.F.);
#4227=ORIENTED_EDGE('',*,*,#3434,.F.);
#4228=ORIENTED_EDGE('',*,*,#3439,.F.);
#4229=ORIENTED_EDGE('',*,*,#3440,.F.);
#4230=ORIENTED_EDGE('',*,*,#3441,.F.);
#4231=ORIENTED_EDGE('',*,*,#3437,.F.);
#4232=ORIENTED_EDGE('',*,*,#3442,.F.);
#4233=ORIENTED_EDGE('',*,*,#3443,.T.);
#4234=ORIENTED_EDGE('',*,*,#3444,.F.);
#4235=ORIENTED_EDGE('',*,*,#3443,.F.);
#4236=ORIENTED_EDGE('',*,*,#3356,.T.);
#4237=ORIENTED_EDGE('',*,*,#3445,.T.);
#4238=ORIENTED_EDGE('',*,*,#3446,.T.);
#4239=ORIENTED_EDGE('',*,*,#3447,.F.);
#4240=ORIENTED_EDGE('',*,*,#3333,.T.);
#4241=ORIENTED_EDGE('',*,*,#3448,.F.);
#4242=ORIENTED_EDGE('',*,*,#3449,.F.);
#4243=ORIENTED_EDGE('',*,*,#3450,.T.);
#4244=ORIENTED_EDGE('',*,*,#3384,.T.);
#4245=ORIENTED_EDGE('',*,*,#3451,.T.);
#4246=ORIENTED_EDGE('',*,*,#3449,.T.);
#4247=ORIENTED_EDGE('',*,*,#3452,.F.);
#4248=ORIENTED_EDGE('',*,*,#3361,.T.);
#4249=ORIENTED_EDGE('',*,*,#3453,.F.);
#4250=ORIENTED_EDGE('',*,*,#3454,.F.);
#4251=ORIENTED_EDGE('',*,*,#3455,.T.);
#4252=ORIENTED_EDGE('',*,*,#3412,.T.);
#4253=ORIENTED_EDGE('',*,*,#3456,.T.);
#4254=ORIENTED_EDGE('',*,*,#3454,.T.);
#4255=ORIENTED_EDGE('',*,*,#3457,.F.);
#4256=ORIENTED_EDGE('',*,*,#3389,.T.);
#4257=ORIENTED_EDGE('',*,*,#3458,.F.);
#4258=ORIENTED_EDGE('',*,*,#3459,.F.);
#4259=ORIENTED_EDGE('',*,*,#3460,.T.);
#4260=ORIENTED_EDGE('',*,*,#3440,.T.);
#4261=ORIENTED_EDGE('',*,*,#3461,.T.);
#4262=ORIENTED_EDGE('',*,*,#3459,.T.);
#4263=ORIENTED_EDGE('',*,*,#3462,.F.);
#4264=ORIENTED_EDGE('',*,*,#3417,.T.);
#4265=ORIENTED_EDGE('',*,*,#3463,.F.);
#4266=ORIENTED_EDGE('',*,*,#3446,.F.);
#4267=ORIENTED_EDGE('',*,*,#3464,.T.);
#4268=ORIENTED_EDGE('',*,*,#3332,.T.);
#4269=ORIENTED_EDGE('',*,*,#3336,.T.);
#4270=ORIENTED_EDGE('',*,*,#3339,.T.);
#4271=ORIENTED_EDGE('',*,*,#3342,.T.);
#4272=ORIENTED_EDGE('',*,*,#3345,.T.);
#4273=ORIENTED_EDGE('',*,*,#3348,.T.);
#4274=ORIENTED_EDGE('',*,*,#3351,.T.);
#4275=ORIENTED_EDGE('',*,*,#3354,.T.);
#4276=ORIENTED_EDGE('',*,*,#3357,.T.);
#4277=ORIENTED_EDGE('',*,*,#3447,.T.);
#4278=ORIENTED_EDGE('',*,*,#3463,.T.);
#4279=ORIENTED_EDGE('',*,*,#3416,.T.);
#4280=ORIENTED_EDGE('',*,*,#3420,.T.);
#4281=ORIENTED_EDGE('',*,*,#3423,.T.);
#4282=ORIENTED_EDGE('',*,*,#3426,.T.);
#4283=ORIENTED_EDGE('',*,*,#3429,.T.);
#4284=ORIENTED_EDGE('',*,*,#3432,.T.);
#4285=ORIENTED_EDGE('',*,*,#3435,.T.);
#4286=ORIENTED_EDGE('',*,*,#3438,.T.);
#4287=ORIENTED_EDGE('',*,*,#3441,.T.);
#4288=ORIENTED_EDGE('',*,*,#3462,.T.);
#4289=ORIENTED_EDGE('',*,*,#3458,.T.);
#4290=ORIENTED_EDGE('',*,*,#3388,.T.);
#4291=ORIENTED_EDGE('',*,*,#3392,.T.);
#4292=ORIENTED_EDGE('',*,*,#3395,.T.);
#4293=ORIENTED_EDGE('',*,*,#3398,.T.);
#4294=ORIENTED_EDGE('',*,*,#3401,.T.);
#4295=ORIENTED_EDGE('',*,*,#3404,.T.);
#4296=ORIENTED_EDGE('',*,*,#3407,.T.);
#4297=ORIENTED_EDGE('',*,*,#3410,.T.);
#4298=ORIENTED_EDGE('',*,*,#3413,.T.);
#4299=ORIENTED_EDGE('',*,*,#3457,.T.);
#4300=ORIENTED_EDGE('',*,*,#3453,.T.);
#4301=ORIENTED_EDGE('',*,*,#3360,.T.);
#4302=ORIENTED_EDGE('',*,*,#3364,.T.);
#4303=ORIENTED_EDGE('',*,*,#3367,.T.);
#4304=ORIENTED_EDGE('',*,*,#3370,.T.);
#4305=ORIENTED_EDGE('',*,*,#3373,.T.);
#4306=ORIENTED_EDGE('',*,*,#3376,.T.);
#4307=ORIENTED_EDGE('',*,*,#3379,.T.);
#4308=ORIENTED_EDGE('',*,*,#3382,.T.);
#4309=ORIENTED_EDGE('',*,*,#3385,.T.);
#4310=ORIENTED_EDGE('',*,*,#3452,.T.);
#4311=ORIENTED_EDGE('',*,*,#3448,.T.);
#4312=ORIENTED_EDGE('',*,*,#3444,.T.);
#4313=ORIENTED_EDGE('',*,*,#3330,.T.);
#4314=ORIENTED_EDGE('',*,*,#3450,.F.);
#4315=ORIENTED_EDGE('',*,*,#3451,.F.);
#4316=ORIENTED_EDGE('',*,*,#3383,.T.);
#4317=ORIENTED_EDGE('',*,*,#3380,.T.);
#4318=ORIENTED_EDGE('',*,*,#3377,.T.);
#4319=ORIENTED_EDGE('',*,*,#3374,.T.);
#4320=ORIENTED_EDGE('',*,*,#3371,.T.);
#4321=ORIENTED_EDGE('',*,*,#3368,.T.);
#4322=ORIENTED_EDGE('',*,*,#3365,.T.);
#4323=ORIENTED_EDGE('',*,*,#3362,.T.);
#4324=ORIENTED_EDGE('',*,*,#3358,.T.);
#4325=ORIENTED_EDGE('',*,*,#3455,.F.);
#4326=ORIENTED_EDGE('',*,*,#3456,.F.);
#4327=ORIENTED_EDGE('',*,*,#3411,.T.);
#4328=ORIENTED_EDGE('',*,*,#3408,.T.);
#4329=ORIENTED_EDGE('',*,*,#3405,.T.);
#4330=ORIENTED_EDGE('',*,*,#3402,.T.);
#4331=ORIENTED_EDGE('',*,*,#3399,.T.);
#4332=ORIENTED_EDGE('',*,*,#3396,.T.);
#4333=ORIENTED_EDGE('',*,*,#3393,.T.);
#4334=ORIENTED_EDGE('',*,*,#3390,.T.);
#4335=ORIENTED_EDGE('',*,*,#3386,.T.);
#4336=ORIENTED_EDGE('',*,*,#3460,.F.);
#4337=ORIENTED_EDGE('',*,*,#3461,.F.);
#4338=ORIENTED_EDGE('',*,*,#3439,.T.);
#4339=ORIENTED_EDGE('',*,*,#3436,.T.);
#4340=ORIENTED_EDGE('',*,*,#3433,.T.);
#4341=ORIENTED_EDGE('',*,*,#3430,.T.);
#4342=ORIENTED_EDGE('',*,*,#3427,.T.);
#4343=ORIENTED_EDGE('',*,*,#3424,.T.);
#4344=ORIENTED_EDGE('',*,*,#3421,.T.);
#4345=ORIENTED_EDGE('',*,*,#3418,.T.);
#4346=ORIENTED_EDGE('',*,*,#3414,.T.);
#4347=ORIENTED_EDGE('',*,*,#3464,.F.);
#4348=ORIENTED_EDGE('',*,*,#3445,.F.);
#4349=ORIENTED_EDGE('',*,*,#3355,.T.);
#4350=ORIENTED_EDGE('',*,*,#3352,.T.);
#4351=ORIENTED_EDGE('',*,*,#3349,.T.);
#4352=ORIENTED_EDGE('',*,*,#3346,.T.);
#4353=ORIENTED_EDGE('',*,*,#3343,.T.);
#4354=ORIENTED_EDGE('',*,*,#3340,.T.);
#4355=ORIENTED_EDGE('',*,*,#3337,.T.);
#4356=ORIENTED_EDGE('',*,*,#3334,.T.);
#4357=ORIENTED_EDGE('',*,*,#3442,.T.);
#5604=PLANE('',#6737);
#5605=PLANE('',#6738);
#5606=PLANE('',#6739);
#5607=PLANE('',#6740);
#5608=PLANE('',#6741);
#5609=PLANE('',#6742);
#5610=PLANE('',#6743);
#5611=PLANE('',#6744);
#5612=PLANE('',#6745);
#5613=PLANE('',#6746);
#5614=PLANE('',#6747);
#5615=PLANE('',#6748);
#5616=PLANE('',#6749);
#5617=PLANE('',#6750);
#5618=PLANE('',#6751);
#5619=PLANE('',#6752);
#5620=PLANE('',#6753);
#5621=PLANE('',#6754);
#5622=PLANE('',#6755);
#5623=PLANE('',#6756);
#5624=PLANE('',#6757);
#5625=PLANE('',#6758);
#5626=PLANE('',#6759);
#5627=PLANE('',#6760);
#5628=PLANE('',#6761);
#5629=PLANE('',#6762);
#5630=PLANE('',#6763);
#5631=PLANE('',#6764);
#5632=PLANE('',#6765);
#5633=PLANE('',#6766);
#5634=PLANE('',#6767);
#5635=PLANE('',#6768);
#5636=PLANE('',#6769);
#5637=PLANE('',#6770);
#5638=PLANE('',#6771);
#5639=PLANE('',#6772);
#5640=PLANE('',#6776);
#5641=PLANE('',#6777);
#5642=PLANE('',#6778);
#5643=PLANE('',#6779);
#5644=PLANE('',#6780);
#5645=PLANE('',#6781);
#5646=PLANE('',#6782);
#5647=PLANE('',#6783);
#5648=PLANE('',#6784);
#5649=PLANE('',#6785);
#5838=ADVANCED_FACE('',(#1038),#5604,.F.);
#5839=ADVANCED_FACE('',(#1039),#5605,.F.);
#5840=ADVANCED_FACE('',(#1040),#5606,.F.);
#5841=ADVANCED_FACE('',(#1041),#5607,.F.);
#5842=ADVANCED_FACE('',(#1042),#5608,.F.);
#5843=ADVANCED_FACE('',(#1043),#5609,.F.);
#5844=ADVANCED_FACE('',(#1044),#5610,.F.);
#5845=ADVANCED_FACE('',(#1045),#5611,.F.);
#5846=ADVANCED_FACE('',(#1046),#5612,.F.);
#5847=ADVANCED_FACE('',(#1047),#5613,.F.);
#5848=ADVANCED_FACE('',(#1048),#5614,.F.);
#5849=ADVANCED_FACE('',(#1049),#5615,.F.);
#5850=ADVANCED_FACE('',(#1050),#5616,.F.);
#5851=ADVANCED_FACE('',(#1051),#5617,.F.);
#5852=ADVANCED_FACE('',(#1052),#5618,.F.);
#5853=ADVANCED_FACE('',(#1053),#5619,.F.);
#5854=ADVANCED_FACE('',(#1054),#5620,.F.);
#5855=ADVANCED_FACE('',(#1055),#5621,.F.);
#5856=ADVANCED_FACE('',(#1056),#5622,.F.);
#5857=ADVANCED_FACE('',(#1057),#5623,.F.);
#5858=ADVANCED_FACE('',(#1058),#5624,.F.);
#5859=ADVANCED_FACE('',(#1059),#5625,.F.);
#5860=ADVANCED_FACE('',(#1060),#5626,.F.);
#5861=ADVANCED_FACE('',(#1061),#5627,.F.);
#5862=ADVANCED_FACE('',(#1062),#5628,.F.);
#5863=ADVANCED_FACE('',(#1063),#5629,.F.);
#5864=ADVANCED_FACE('',(#1064),#5630,.F.);
#5865=ADVANCED_FACE('',(#1065),#5631,.F.);
#5866=ADVANCED_FACE('',(#1066),#5632,.F.);
#5867=ADVANCED_FACE('',(#1067),#5633,.F.);
#5868=ADVANCED_FACE('',(#1068),#5634,.F.);
#5869=ADVANCED_FACE('',(#1069),#5635,.F.);
#5870=ADVANCED_FACE('',(#1070),#5636,.F.);
#5871=ADVANCED_FACE('',(#1071),#5637,.F.);
#5872=ADVANCED_FACE('',(#1072),#5638,.F.);
#5873=ADVANCED_FACE('',(#1073),#5639,.F.);
#5874=ADVANCED_FACE('',(#1074),#938,.F.);
#5875=ADVANCED_FACE('',(#1075),#5640,.T.);
#5876=ADVANCED_FACE('',(#1076),#5641,.T.);
#5877=ADVANCED_FACE('',(#1077),#5642,.T.);
#5878=ADVANCED_FACE('',(#1078),#5643,.T.);
#5879=ADVANCED_FACE('',(#1079),#5644,.T.);
#5880=ADVANCED_FACE('',(#1080),#5645,.T.);
#5881=ADVANCED_FACE('',(#1081),#5646,.T.);
#5882=ADVANCED_FACE('',(#1082),#5647,.T.);
#5883=ADVANCED_FACE('',(#1083,#562),#5648,.T.);
#5884=ADVANCED_FACE('',(#1084,#563),#5649,.F.);
#6206=CLOSED_SHELL('',(#5838,#5839,#5840,#5841,#5842,#5843,#5844,#5845,
#5846,#5847,#5848,#5849,#5850,#5851,#5852,#5853,#5854,#5855,#5856,#5857,
#5858,#5859,#5860,#5861,#5862,#5863,#5864,#5865,#5866,#5867,#5868,#5869,
#5870,#5871,#5872,#5873,#5874,#5875,#5876,#5877,#5878,#5879,#5880,#5881,
#5882,#5883,#5884));
#6736=AXIS2_PLACEMENT_3D('',#9477,#7496,#7497);
#6737=AXIS2_PLACEMENT_3D('',#9478,#7498,#7499);
#6738=AXIS2_PLACEMENT_3D('',#9487,#7504,#7505);
#6739=AXIS2_PLACEMENT_3D('',#9493,#7509,#7510);
#6740=AXIS2_PLACEMENT_3D('',#9499,#7514,#7515);
#6741=AXIS2_PLACEMENT_3D('',#9505,#7519,#7520);
#6742=AXIS2_PLACEMENT_3D('',#9511,#7524,#7525);
#6743=AXIS2_PLACEMENT_3D('',#9517,#7529,#7530);
#6744=AXIS2_PLACEMENT_3D('',#9523,#7534,#7535);
#6745=AXIS2_PLACEMENT_3D('',#9529,#7539,#7540);
#6746=AXIS2_PLACEMENT_3D('',#9535,#7544,#7545);
#6747=AXIS2_PLACEMENT_3D('',#9544,#7550,#7551);
#6748=AXIS2_PLACEMENT_3D('',#9550,#7555,#7556);
#6749=AXIS2_PLACEMENT_3D('',#9556,#7560,#7561);
#6750=AXIS2_PLACEMENT_3D('',#9562,#7565,#7566);
#6751=AXIS2_PLACEMENT_3D('',#9568,#7570,#7571);
#6752=AXIS2_PLACEMENT_3D('',#9574,#7575,#7576);
#6753=AXIS2_PLACEMENT_3D('',#9580,#7580,#7581);
#6754=AXIS2_PLACEMENT_3D('',#9586,#7585,#7586);
#6755=AXIS2_PLACEMENT_3D('',#9592,#7590,#7591);
#6756=AXIS2_PLACEMENT_3D('',#9601,#7596,#7597);
#6757=AXIS2_PLACEMENT_3D('',#9607,#7601,#7602);
#6758=AXIS2_PLACEMENT_3D('',#9613,#7606,#7607);
#6759=AXIS2_PLACEMENT_3D('',#9619,#7611,#7612);
#6760=AXIS2_PLACEMENT_3D('',#9625,#7616,#7617);
#6761=AXIS2_PLACEMENT_3D('',#9631,#7621,#7622);
#6762=AXIS2_PLACEMENT_3D('',#9637,#7626,#7627);
#6763=AXIS2_PLACEMENT_3D('',#9643,#7631,#7632);
#6764=AXIS2_PLACEMENT_3D('',#9649,#7636,#7637);
#6765=AXIS2_PLACEMENT_3D('',#9658,#7642,#7643);
#6766=AXIS2_PLACEMENT_3D('',#9664,#7647,#7648);
#6767=AXIS2_PLACEMENT_3D('',#9670,#7652,#7653);
#6768=AXIS2_PLACEMENT_3D('',#9676,#7657,#7658);
#6769=AXIS2_PLACEMENT_3D('',#9682,#7662,#7663);
#6770=AXIS2_PLACEMENT_3D('',#9688,#7667,#7668);
#6771=AXIS2_PLACEMENT_3D('',#9694,#7672,#7673);
#6772=AXIS2_PLACEMENT_3D('',#9700,#7677,#7678);
#6773=AXIS2_PLACEMENT_3D('',#9706,#7682,#7683);
#6774=AXIS2_PLACEMENT_3D('',#9708,#7684,#7685);
#6775=AXIS2_PLACEMENT_3D('',#9711,#7687,#7688);
#6776=AXIS2_PLACEMENT_3D('',#9712,#7689,#7690);
#6777=AXIS2_PLACEMENT_3D('',#9718,#7694,#7695);
#6778=AXIS2_PLACEMENT_3D('',#9724,#7699,#7700);
#6779=AXIS2_PLACEMENT_3D('',#9727,#7703,#7704);
#6780=AXIS2_PLACEMENT_3D('',#9733,#7708,#7709);
#6781=AXIS2_PLACEMENT_3D('',#9736,#7712,#7713);
#6782=AXIS2_PLACEMENT_3D('',#9742,#7717,#7718);
#6783=AXIS2_PLACEMENT_3D('',#9745,#7721,#7722);
#6784=AXIS2_PLACEMENT_3D('',#9748,#7725,#7726);
#6785=AXIS2_PLACEMENT_3D('',#9749,#7727,#7728);
#7496=DIRECTION('axis',(0.,0.,1.));
#7497=DIRECTION('refdir',(1.,0.,0.));
#7498=DIRECTION('center_axis',(0.,0.,-1.));
#7499=DIRECTION('ref_axis',(0.,1.,0.));
#7500=DIRECTION('',(0.,1.,0.));
#7501=DIRECTION('',(1.,0.,0.));
#7502=DIRECTION('',(0.,-1.,0.));
#7503=DIRECTION('',(1.,0.,0.));
#7504=DIRECTION('center_axis',(0.,1.,-8.88178419700125E-16));
#7505=DIRECTION('ref_axis',(0.,8.88178419700125E-16,1.));
#7506=DIRECTION('',(0.,8.88178419700125E-16,1.));
#7507=DIRECTION('',(1.,0.,0.));
#7508=DIRECTION('',(0.,-8.88178419700125E-16,-1.));
#7509=DIRECTION('center_axis',(0.,-7.40148683083439E-16,-1.));
#7510=DIRECTION('ref_axis',(0.,1.,-7.40148683083439E-16));
#7511=DIRECTION('',(0.,1.,-7.40148683083439E-16));
#7512=DIRECTION('',(1.,0.,0.));
#7513=DIRECTION('',(0.,-1.,7.40148683083439E-16));
#7514=DIRECTION('center_axis',(0.,-0.707106781186547,-0.707106781186548));
#7515=DIRECTION('ref_axis',(0.,0.707106781186548,-0.707106781186547));
#7516=DIRECTION('',(0.,0.707106781186548,-0.707106781186547));
#7517=DIRECTION('',(1.,0.,0.));
#7518=DIRECTION('',(0.,-0.707106781186548,0.707106781186547));
#7519=DIRECTION('center_axis',(0.,-1.,2.77555756156289E-16));
#7520=DIRECTION('ref_axis',(0.,-2.77555756156289E-16,-1.));
#7521=DIRECTION('',(0.,-2.77555756156289E-16,-1.));
#7522=DIRECTION('',(1.,0.,0.));
#7523=DIRECTION('',(0.,2.77555756156289E-16,1.));
#7524=DIRECTION('center_axis',(0.,-0.707106781186547,0.707106781186548));
#7525=DIRECTION('ref_axis',(0.,-0.707106781186548,-0.707106781186547));
#7526=DIRECTION('',(0.,-0.707106781186548,-0.707106781186547));
#7527=DIRECTION('',(1.,0.,0.));
#7528=DIRECTION('',(0.,0.707106781186548,0.707106781186547));
#7529=DIRECTION('center_axis',(0.,7.40148683083438E-16,1.));
#7530=DIRECTION('ref_axis',(0.,-1.,7.40148683083438E-16));
#7531=DIRECTION('',(0.,-1.,7.40148683083438E-16));
#7532=DIRECTION('',(1.,0.,0.));
#7533=DIRECTION('',(0.,1.,-7.40148683083438E-16));
#7534=DIRECTION('center_axis',(0.,1.,-4.44089209850063E-16));
#7535=DIRECTION('ref_axis',(0.,4.44089209850063E-16,1.));
#7536=DIRECTION('',(0.,4.44089209850063E-16,1.));
#7537=DIRECTION('',(1.,0.,0.));
#7538=DIRECTION('',(0.,-4.44089209850063E-16,-1.));
#7539=DIRECTION('center_axis',(0.,2.41352831440251E-16,1.));
#7540=DIRECTION('ref_axis',(0.,-1.,2.41352831440251E-16));
#7541=DIRECTION('',(0.,-1.,2.41352831440251E-16));
#7542=DIRECTION('',(-1.,0.,0.));
#7543=DIRECTION('',(0.,1.,-2.41352831440251E-16));
#7544=DIRECTION('center_axis',(0.,-1.,2.41352831440251E-16));
#7545=DIRECTION('ref_axis',(0.,-2.41352831440251E-16,-1.));
#7546=DIRECTION('',(0.,-2.41352831440251E-16,-1.));
#7547=DIRECTION('',(1.,0.,0.));
#7548=DIRECTION('',(0.,2.41352831440251E-16,1.));
#7549=DIRECTION('',(1.,0.,0.));
#7550=DIRECTION('center_axis',(0.,0.,-1.));
#7551=DIRECTION('ref_axis',(0.,1.,0.));
#7552=DIRECTION('',(0.,1.,0.));
#7553=DIRECTION('',(1.,0.,0.));
#7554=DIRECTION('',(0.,-1.,0.));
#7555=DIRECTION('center_axis',(0.,-1.,0.));
#7556=DIRECTION('ref_axis',(0.,0.,-1.));
#7557=DIRECTION('',(0.,0.,-1.));
#7558=DIRECTION('',(1.,0.,0.));
#7559=DIRECTION('',(0.,0.,1.));
#7560=DIRECTION('center_axis',(0.,-0.707106781186547,0.707106781186548));
#7561=DIRECTION('ref_axis',(0.,-0.707106781186548,-0.707106781186547));
#7562=DIRECTION('',(0.,-0.707106781186548,-0.707106781186547));
#7563=DIRECTION('',(1.,0.,0.));
#7564=DIRECTION('',(0.,0.707106781186548,0.707106781186547));
#7565=DIRECTION('center_axis',(0.,0.,1.));
#7566=DIRECTION('ref_axis',(0.,-1.,0.));
#7567=DIRECTION('',(0.,-1.,0.));
#7568=DIRECTION('',(1.,0.,0.));
#7569=DIRECTION('',(0.,1.,0.));
#7570=DIRECTION('center_axis',(0.,0.707106781186548,0.707106781186547));
#7571=DIRECTION('ref_axis',(0.,-0.707106781186547,0.707106781186548));
#7572=DIRECTION('',(0.,-0.707106781186547,0.707106781186548));
#7573=DIRECTION('',(1.,0.,0.));
#7574=DIRECTION('',(0.,0.707106781186547,-0.707106781186548));
#7575=DIRECTION('center_axis',(0.,1.,0.));
#7576=DIRECTION('ref_axis',(0.,0.,1.));
#7577=DIRECTION('',(0.,0.,1.));
#7578=DIRECTION('',(1.,0.,0.));
#7579=DIRECTION('',(0.,0.,-1.));
#7580=DIRECTION('center_axis',(0.,0.,-1.));
#7581=DIRECTION('ref_axis',(0.,1.,0.));
#7582=DIRECTION('',(0.,1.,0.));
#7583=DIRECTION('',(1.,0.,0.));
#7584=DIRECTION('',(0.,-1.,0.));
#7585=DIRECTION('center_axis',(0.,1.,-2.41352831440251E-16));
#7586=DIRECTION('ref_axis',(0.,2.41352831440251E-16,1.));
#7587=DIRECTION('',(0.,2.41352831440251E-16,1.));
#7588=DIRECTION('',(-1.,0.,0.));
#7589=DIRECTION('',(0.,-2.41352831440251E-16,-1.));
#7590=DIRECTION('center_axis',(0.,0.,1.));
#7591=DIRECTION('ref_axis',(0.,-1.,0.));
#7592=DIRECTION('',(0.,-1.,0.));
#7593=DIRECTION('',(1.,0.,0.));
#7594=DIRECTION('',(0.,1.,0.));
#7595=DIRECTION('',(1.,0.,0.));
#7596=DIRECTION('center_axis',(0.,-1.,0.));
#7597=DIRECTION('ref_axis',(0.,0.,-1.));
#7598=DIRECTION('',(0.,0.,-1.));
#7599=DIRECTION('',(1.,0.,0.));
#7600=DIRECTION('',(0.,0.,1.));
#7601=DIRECTION('center_axis',(0.,0.,1.));
#7602=DIRECTION('ref_axis',(0.,-1.,0.));
#7603=DIRECTION('',(0.,-1.,0.));
#7604=DIRECTION('',(1.,0.,0.));
#7605=DIRECTION('',(0.,1.,0.));
#7606=DIRECTION('center_axis',(0.,0.707106781186548,0.707106781186548));
#7607=DIRECTION('ref_axis',(0.,-0.707106781186548,0.707106781186548));
#7608=DIRECTION('',(0.,-0.707106781186548,0.707106781186548));
#7609=DIRECTION('',(1.,0.,0.));
#7610=DIRECTION('',(0.,0.707106781186548,-0.707106781186548));
#7611=DIRECTION('center_axis',(0.,1.,0.));
#7612=DIRECTION('ref_axis',(0.,0.,1.));
#7613=DIRECTION('',(0.,0.,1.));
#7614=DIRECTION('',(1.,0.,0.));
#7615=DIRECTION('',(0.,0.,-1.));
#7616=DIRECTION('center_axis',(0.,0.707106781186548,-0.707106781186547));
#7617=DIRECTION('ref_axis',(0.,0.707106781186547,0.707106781186548));
#7618=DIRECTION('',(0.,0.707106781186547,0.707106781186548));
#7619=DIRECTION('',(1.,0.,0.));
#7620=DIRECTION('',(0.,-0.707106781186547,-0.707106781186548));
#7621=DIRECTION('center_axis',(0.,-7.40148683083438E-16,-1.));
#7622=DIRECTION('ref_axis',(0.,1.,-7.40148683083438E-16));
#7623=DIRECTION('',(0.,1.,-7.40148683083438E-16));
#7624=DIRECTION('',(1.,0.,0.));
#7625=DIRECTION('',(0.,-1.,7.40148683083438E-16));
#7626=DIRECTION('center_axis',(0.,-1.,0.));
#7627=DIRECTION('ref_axis',(0.,0.,-1.));
#7628=DIRECTION('',(0.,0.,-1.));
#7629=DIRECTION('',(1.,0.,0.));
#7630=DIRECTION('',(0.,0.,1.));
#7631=DIRECTION('center_axis',(0.,0.,-1.));
#7632=DIRECTION('ref_axis',(0.,1.,0.));
#7633=DIRECTION('',(0.,1.,0.));
#7634=DIRECTION('',(-1.,0.,0.));
#7635=DIRECTION('',(0.,-1.,0.));
#7636=DIRECTION('center_axis',(0.,1.,0.));
#7637=DIRECTION('ref_axis',(0.,0.,1.));
#7638=DIRECTION('',(0.,0.,1.));
#7639=DIRECTION('',(1.,0.,0.));
#7640=DIRECTION('',(0.,0.,-1.));
#7641=DIRECTION('',(1.,0.,0.));
#7642=DIRECTION('center_axis',(0.,0.,1.));
#7643=DIRECTION('ref_axis',(0.,-1.,0.));
#7644=DIRECTION('',(0.,-1.,0.));
#7645=DIRECTION('',(1.,0.,0.));
#7646=DIRECTION('',(0.,1.,0.));
#7647=DIRECTION('center_axis',(0.,1.,0.));
#7648=DIRECTION('ref_axis',(0.,0.,1.));
#7649=DIRECTION('',(0.,0.,1.));
#7650=DIRECTION('',(1.,0.,0.));
#7651=DIRECTION('',(0.,0.,-1.));
#7652=DIRECTION('center_axis',(0.,0.707106781186547,-0.707106781186548));
#7653=DIRECTION('ref_axis',(0.,0.707106781186548,0.707106781186547));
#7654=DIRECTION('',(0.,0.707106781186548,0.707106781186547));
#7655=DIRECTION('',(1.,0.,0.));
#7656=DIRECTION('',(0.,-0.707106781186548,-0.707106781186547));
#7657=DIRECTION('center_axis',(0.,0.,-1.));
#7658=DIRECTION('ref_axis',(0.,1.,0.));
#7659=DIRECTION('',(0.,1.,0.));
#7660=DIRECTION('',(1.,0.,0.));
#7661=DIRECTION('',(0.,-1.,0.));
#7662=DIRECTION('center_axis',(0.,-0.707106781186547,-0.707106781186548));
#7663=DIRECTION('ref_axis',(0.,0.707106781186548,-0.707106781186547));
#7664=DIRECTION('',(0.,0.707106781186548,-0.707106781186547));
#7665=DIRECTION('',(1.,0.,0.));
#7666=DIRECTION('',(0.,-0.707106781186548,0.707106781186547));
#7667=DIRECTION('center_axis',(0.,-1.,0.));
#7668=DIRECTION('ref_axis',(0.,0.,-1.));
#7669=DIRECTION('',(0.,0.,-1.));
#7670=DIRECTION('',(1.,0.,0.));
#7671=DIRECTION('',(0.,0.,1.));
#7672=DIRECTION('center_axis',(0.,0.,1.));
#7673=DIRECTION('ref_axis',(0.,-1.,0.));
#7674=DIRECTION('',(0.,-1.,0.));
#7675=DIRECTION('',(1.,0.,0.));
#7676=DIRECTION('',(0.,1.,0.));
#7677=DIRECTION('center_axis',(0.,-1.,0.));
#7678=DIRECTION('ref_axis',(0.,0.,-1.));
#7679=DIRECTION('',(0.,0.,-1.));
#7680=DIRECTION('',(-1.,0.,0.));
#7681=DIRECTION('',(0.,0.,1.));
#7682=DIRECTION('center_axis',(1.,0.,0.));
#7683=DIRECTION('ref_axis',(0.,0.,-1.));
#7684=DIRECTION('center_axis',(1.,0.,0.));
#7685=DIRECTION('ref_axis',(0.,0.,-1.));
#7686=DIRECTION('',(1.,0.,0.));
#7687=DIRECTION('center_axis',(-1.,0.,0.));
#7688=DIRECTION('ref_axis',(0.,0.,-1.));
#7689=DIRECTION('center_axis',(0.,1.,0.));
#7690=DIRECTION('ref_axis',(0.,0.,1.));
#7691=DIRECTION('',(0.,0.,1.));
#7692=DIRECTION('',(1.,0.,0.));
#7693=DIRECTION('',(0.,0.,1.));
#7694=DIRECTION('center_axis',(0.,1.,0.));
#7695=DIRECTION('ref_axis',(0.,0.,1.));
#7696=DIRECTION('',(0.,0.,1.));
#7697=DIRECTION('',(1.,0.,0.));
#7698=DIRECTION('',(0.,0.,1.));
#7699=DIRECTION('center_axis',(0.,0.,-1.));
#7700=DIRECTION('ref_axis',(0.,1.,0.));
#7701=DIRECTION('',(0.,1.,0.));
#7702=DIRECTION('',(0.,1.,0.));
#7703=DIRECTION('center_axis',(0.,0.,-1.));
#7704=DIRECTION('ref_axis',(0.,1.,0.));
#7705=DIRECTION('',(0.,1.,0.));
#7706=DIRECTION('',(1.,0.,0.));
#7707=DIRECTION('',(0.,1.,0.));
#7708=DIRECTION('center_axis',(0.,-1.,0.));
#7709=DIRECTION('ref_axis',(0.,0.,-1.));
#7710=DIRECTION('',(0.,0.,-1.));
#7711=DIRECTION('',(0.,0.,-1.));
#7712=DIRECTION('center_axis',(0.,-1.,0.));
#7713=DIRECTION('ref_axis',(0.,0.,-1.));
#7714=DIRECTION('',(0.,0.,-1.));
#7715=DIRECTION('',(1.,0.,0.));
#7716=DIRECTION('',(0.,0.,-1.));
#7717=DIRECTION('center_axis',(0.,0.,1.));
#7718=DIRECTION('ref_axis',(0.,-1.,0.));
#7719=DIRECTION('',(0.,-1.,0.));
#7720=DIRECTION('',(0.,-1.,0.));
#7721=DIRECTION('center_axis',(0.,0.,1.));
#7722=DIRECTION('ref_axis',(0.,-1.,0.));
#7723=DIRECTION('',(0.,-1.,0.));
#7724=DIRECTION('',(0.,-1.,0.));
#7725=DIRECTION('center_axis',(1.,0.,0.));
#7726=DIRECTION('ref_axis',(0.,0.,-1.));
#7727=DIRECTION('center_axis',(1.,0.,0.));
#7728=DIRECTION('ref_axis',(0.,0.,-1.));
#9477=CARTESIAN_POINT('',(0.,0.,0.));
#9478=CARTESIAN_POINT('Origin',(-0.1,0.82,-0.3));
#9479=CARTESIAN_POINT('',(0.,0.82,-0.3));
#9480=CARTESIAN_POINT('',(0.,1.,-0.3));
#9481=CARTESIAN_POINT('',(0.,0.41,-0.3));
#9482=CARTESIAN_POINT('',(40.,0.82,-0.3));
#9483=CARTESIAN_POINT('',(-0.1,0.82,-0.3));
#9484=CARTESIAN_POINT('',(40.,1.,-0.3));
#9485=CARTESIAN_POINT('',(40.,0.41,-0.3));
#9486=CARTESIAN_POINT('',(-0.05,1.,-0.3));
#9487=CARTESIAN_POINT('Origin',(-0.1,0.82,-0.55));
#9488=CARTESIAN_POINT('',(0.,0.82,-0.55));
#9489=CARTESIAN_POINT('',(0.,0.82,-0.275));
#9490=CARTESIAN_POINT('',(40.,0.82,-0.55));
#9491=CARTESIAN_POINT('',(-0.1,0.82,-0.55));
#9492=CARTESIAN_POINT('',(40.,0.82,-0.275));
#9493=CARTESIAN_POINT('Origin',(-0.1,0.67,-0.55));
#9494=CARTESIAN_POINT('',(0.,0.67,-0.55));
#9495=CARTESIAN_POINT('',(0.,0.335,-0.55));
#9496=CARTESIAN_POINT('',(40.,0.67,-0.55));
#9497=CARTESIAN_POINT('',(-0.1,0.67,-0.55));
#9498=CARTESIAN_POINT('',(40.,0.335,-0.55));
#9499=CARTESIAN_POINT('Origin',(-0.1,0.42,-0.3));
#9500=CARTESIAN_POINT('',(0.,0.42,-0.3));
#9501=CARTESIAN_POINT('',(0.,0.24,-0.12));
#9502=CARTESIAN_POINT('',(40.,0.42,-0.3));
#9503=CARTESIAN_POINT('',(-0.1,0.42,-0.3));
#9504=CARTESIAN_POINT('',(40.,0.24,-0.12));
#9505=CARTESIAN_POINT('Origin',(-0.1,0.42,0.3));
#9506=CARTESIAN_POINT('',(0.,0.42,0.3));
#9507=CARTESIAN_POINT('',(0.,0.42,0.15));
#9508=CARTESIAN_POINT('',(40.,0.42,0.3));
#9509=CARTESIAN_POINT('',(-0.1,0.42,0.3));
#9510=CARTESIAN_POINT('',(40.,0.42,0.15));
#9511=CARTESIAN_POINT('Origin',(-0.1,0.67,0.55));
#9512=CARTESIAN_POINT('',(0.,0.67,0.55));
#9513=CARTESIAN_POINT('',(6.93889390390723E-18,0.365,0.245));
#9514=CARTESIAN_POINT('',(40.,0.67,0.55));
#9515=CARTESIAN_POINT('',(-0.1,0.67,0.55));
#9516=CARTESIAN_POINT('',(40.,0.365,0.245));
#9517=CARTESIAN_POINT('Origin',(-0.1,0.82,0.55));
#9518=CARTESIAN_POINT('',(0.,0.82,0.55));
#9519=CARTESIAN_POINT('',(0.,0.41,0.55));
#9520=CARTESIAN_POINT('',(40.,0.82,0.55));
#9521=CARTESIAN_POINT('',(-0.1,0.82,0.55));
#9522=CARTESIAN_POINT('',(40.,0.41,0.55));
#9523=CARTESIAN_POINT('Origin',(-0.1,0.82,0.3));
#9524=CARTESIAN_POINT('',(0.,0.82,0.3));
#9525=CARTESIAN_POINT('',(0.,0.82,0.15));
#9526=CARTESIAN_POINT('',(40.,0.82,0.3));
#9527=CARTESIAN_POINT('',(-0.1,0.82,0.3));
#9528=CARTESIAN_POINT('',(40.,0.82,0.15));
#9529=CARTESIAN_POINT('Origin',(-0.1,1.05,0.3));
#9530=CARTESIAN_POINT('',(0.,1.,0.3));
#9531=CARTESIAN_POINT('',(0.,0.525,0.3));
#9532=CARTESIAN_POINT('',(40.,1.,0.3));
#9533=CARTESIAN_POINT('',(-0.05,1.,0.3));
#9534=CARTESIAN_POINT('',(40.,0.525,0.3));
#9535=CARTESIAN_POINT('Origin',(-0.1,-0.3,-0.82));
#9536=CARTESIAN_POINT('',(0.,-0.3,-0.82));
#9537=CARTESIAN_POINT('',(0.,-0.3,-1.));
#9538=CARTESIAN_POINT('',(0.,-0.3,-0.41));
#9539=CARTESIAN_POINT('',(40.,-0.3,-0.82));
#9540=CARTESIAN_POINT('',(-0.1,-0.3,-0.82));
#9541=CARTESIAN_POINT('',(40.,-0.3,-1.));
#9542=CARTESIAN_POINT('',(40.,-0.3,-0.41));
#9543=CARTESIAN_POINT('',(-0.05,-0.3,-1.));
#9544=CARTESIAN_POINT('Origin',(-0.1,-0.55,-0.82));
#9545=CARTESIAN_POINT('',(0.,-0.55,-0.82));
#9546=CARTESIAN_POINT('',(0.,-0.275,-0.82));
#9547=CARTESIAN_POINT('',(40.,-0.55,-0.82));
#9548=CARTESIAN_POINT('',(-0.1,-0.55,-0.82));
#9549=CARTESIAN_POINT('',(40.,-0.275,-0.82));
#9550=CARTESIAN_POINT('Origin',(-0.1,-0.55,-0.67));
#9551=CARTESIAN_POINT('',(0.,-0.55,-0.67));
#9552=CARTESIAN_POINT('',(0.,-0.55,-0.335));
#9553=CARTESIAN_POINT('',(40.,-0.55,-0.67));
#9554=CARTESIAN_POINT('',(-0.1,-0.55,-0.67));
#9555=CARTESIAN_POINT('',(40.,-0.55,-0.335));
#9556=CARTESIAN_POINT('Origin',(-0.1,-0.3,-0.42));
#9557=CARTESIAN_POINT('',(0.,-0.3,-0.42));
#9558=CARTESIAN_POINT('',(0.,-0.12,-0.24));
#9559=CARTESIAN_POINT('',(40.,-0.3,-0.42));
#9560=CARTESIAN_POINT('',(-0.1,-0.3,-0.42));
#9561=CARTESIAN_POINT('',(40.,-0.12,-0.24));
#9562=CARTESIAN_POINT('Origin',(-0.1,0.3,-0.42));
#9563=CARTESIAN_POINT('',(0.,0.3,-0.42));
#9564=CARTESIAN_POINT('',(0.,0.15,-0.42));
#9565=CARTESIAN_POINT('',(40.,0.3,-0.42));
#9566=CARTESIAN_POINT('',(-0.1,0.3,-0.42));
#9567=CARTESIAN_POINT('',(40.,0.15,-0.42));
#9568=CARTESIAN_POINT('Origin',(-0.1,0.55,-0.67));
#9569=CARTESIAN_POINT('',(0.,0.55,-0.67));
#9570=CARTESIAN_POINT('',(0.,0.245,-0.365));
#9571=CARTESIAN_POINT('',(40.,0.55,-0.67));
#9572=CARTESIAN_POINT('',(-0.1,0.55,-0.67));
#9573=CARTESIAN_POINT('',(40.,0.245,-0.365));
#9574=CARTESIAN_POINT('Origin',(-0.1,0.55,-0.82));
#9575=CARTESIAN_POINT('',(0.,0.55,-0.82));
#9576=CARTESIAN_POINT('',(0.,0.55,-0.41));
#9577=CARTESIAN_POINT('',(40.,0.55,-0.82));
#9578=CARTESIAN_POINT('',(-0.1,0.55,-0.82));
#9579=CARTESIAN_POINT('',(40.,0.55,-0.41));
#9580=CARTESIAN_POINT('Origin',(-0.1,0.3,-0.82));
#9581=CARTESIAN_POINT('',(0.,0.3,-0.82));
#9582=CARTESIAN_POINT('',(0.,0.15,-0.82));
#9583=CARTESIAN_POINT('',(40.,0.3,-0.82));
#9584=CARTESIAN_POINT('',(-0.1,0.3,-0.82));
#9585=CARTESIAN_POINT('',(40.,0.15,-0.82));
#9586=CARTESIAN_POINT('Origin',(-0.1,0.3,-1.05));
#9587=CARTESIAN_POINT('',(0.,0.3,-1.));
#9588=CARTESIAN_POINT('',(0.,0.3,-0.525));
#9589=CARTESIAN_POINT('',(40.,0.3,-1.));
#9590=CARTESIAN_POINT('',(-0.05,0.3,-1.));
#9591=CARTESIAN_POINT('',(40.,0.3,-0.525));
#9592=CARTESIAN_POINT('Origin',(-0.1,-0.82,0.3));
#9593=CARTESIAN_POINT('',(0.,-0.82,0.3));
#9594=CARTESIAN_POINT('',(0.,-1.,0.3));
#9595=CARTESIAN_POINT('',(0.,-0.41,0.3));
#9596=CARTESIAN_POINT('',(40.,-0.82,0.3));
#9597=CARTESIAN_POINT('',(-0.1,-0.82,0.3));
#9598=CARTESIAN_POINT('',(40.,-1.,0.3));
#9599=CARTESIAN_POINT('',(40.,-0.41,0.3));
#9600=CARTESIAN_POINT('',(-0.05,-1.,0.3));
#9601=CARTESIAN_POINT('Origin',(-0.1,-0.82,0.55));
#9602=CARTESIAN_POINT('',(0.,-0.82,0.55));
#9603=CARTESIAN_POINT('',(0.,-0.82,0.275));
#9604=CARTESIAN_POINT('',(40.,-0.82,0.55));
#9605=CARTESIAN_POINT('',(-0.1,-0.82,0.55));
#9606=CARTESIAN_POINT('',(40.,-0.82,0.275));
#9607=CARTESIAN_POINT('Origin',(-0.1,-0.67,0.55));
#9608=CARTESIAN_POINT('',(0.,-0.67,0.55));
#9609=CARTESIAN_POINT('',(0.,-0.335,0.55));
#9610=CARTESIAN_POINT('',(40.,-0.67,0.55));
#9611=CARTESIAN_POINT('',(-0.1,-0.67,0.55));
#9612=CARTESIAN_POINT('',(40.,-0.335,0.55));
#9613=CARTESIAN_POINT('Origin',(-0.1,-0.42,0.3));
#9614=CARTESIAN_POINT('',(0.,-0.42,0.3));
#9615=CARTESIAN_POINT('',(-6.93889390390723E-18,-0.24,0.12));
#9616=CARTESIAN_POINT('',(40.,-0.42,0.3));
#9617=CARTESIAN_POINT('',(-0.1,-0.42,0.3));
#9618=CARTESIAN_POINT('',(40.,-0.24,0.12));
#9619=CARTESIAN_POINT('Origin',(-0.1,-0.42,-0.3));
#9620=CARTESIAN_POINT('',(0.,-0.42,-0.3));
#9621=CARTESIAN_POINT('',(0.,-0.42,-0.15));
#9622=CARTESIAN_POINT('',(40.,-0.42,-0.3));
#9623=CARTESIAN_POINT('',(-0.1,-0.42,-0.3));
#9624=CARTESIAN_POINT('',(40.,-0.42,-0.15));
#9625=CARTESIAN_POINT('Origin',(-0.1,-0.67,-0.55));
#9626=CARTESIAN_POINT('',(0.,-0.67,-0.55));
#9627=CARTESIAN_POINT('',(0.,-0.365,-0.245));
#9628=CARTESIAN_POINT('',(40.,-0.67,-0.55));
#9629=CARTESIAN_POINT('',(-0.1,-0.67,-0.55));
#9630=CARTESIAN_POINT('',(40.,-0.365,-0.245));
#9631=CARTESIAN_POINT('Origin',(-0.1,-0.82,-0.55));
#9632=CARTESIAN_POINT('',(0.,-0.82,-0.55));
#9633=CARTESIAN_POINT('',(0.,-0.41,-0.55));
#9634=CARTESIAN_POINT('',(40.,-0.82,-0.55));
#9635=CARTESIAN_POINT('',(-0.1,-0.82,-0.55));
#9636=CARTESIAN_POINT('',(40.,-0.41,-0.55));
#9637=CARTESIAN_POINT('Origin',(-0.1,-0.82,-0.3));
#9638=CARTESIAN_POINT('',(0.,-0.82,-0.3));
#9639=CARTESIAN_POINT('',(0.,-0.82,-0.15));
#9640=CARTESIAN_POINT('',(40.,-0.82,-0.3));
#9641=CARTESIAN_POINT('',(-0.1,-0.82,-0.3));
#9642=CARTESIAN_POINT('',(40.,-0.82,-0.15));
#9643=CARTESIAN_POINT('Origin',(-0.1,-1.05,-0.3));
#9644=CARTESIAN_POINT('',(0.,-1.,-0.3));
#9645=CARTESIAN_POINT('',(0.,-0.525,-0.3));
#9646=CARTESIAN_POINT('',(40.,-1.,-0.3));
#9647=CARTESIAN_POINT('',(-0.05,-1.,-0.3));
#9648=CARTESIAN_POINT('',(40.,-0.525,-0.3));
#9649=CARTESIAN_POINT('Origin',(-0.1,0.3,0.82));
#9650=CARTESIAN_POINT('',(0.,0.3,0.82));
#9651=CARTESIAN_POINT('',(0.,0.3,1.));
#9652=CARTESIAN_POINT('',(0.,0.3,0.41));
#9653=CARTESIAN_POINT('',(40.,0.3,0.82));
#9654=CARTESIAN_POINT('',(-0.1,0.3,0.82));
#9655=CARTESIAN_POINT('',(40.,0.3,1.));
#9656=CARTESIAN_POINT('',(40.,0.3,0.41));
#9657=CARTESIAN_POINT('',(-0.05,0.3,1.));
#9658=CARTESIAN_POINT('Origin',(-0.1,0.55,0.82));
#9659=CARTESIAN_POINT('',(0.,0.55,0.82));
#9660=CARTESIAN_POINT('',(0.,0.275,0.82));
#9661=CARTESIAN_POINT('',(40.,0.55,0.82));
#9662=CARTESIAN_POINT('',(-0.1,0.55,0.82));
#9663=CARTESIAN_POINT('',(40.,0.275,0.82));
#9664=CARTESIAN_POINT('Origin',(-0.1,0.55,0.67));
#9665=CARTESIAN_POINT('',(0.,0.55,0.67));
#9666=CARTESIAN_POINT('',(0.,0.55,0.335));
#9667=CARTESIAN_POINT('',(40.,0.55,0.67));
#9668=CARTESIAN_POINT('',(-0.1,0.55,0.67));
#9669=CARTESIAN_POINT('',(40.,0.55,0.335));
#9670=CARTESIAN_POINT('Origin',(-0.1,0.3,0.42));
#9671=CARTESIAN_POINT('',(0.,0.3,0.42));
#9672=CARTESIAN_POINT('',(6.93889390390723E-18,0.12,0.24));
#9673=CARTESIAN_POINT('',(40.,0.3,0.42));
#9674=CARTESIAN_POINT('',(-0.1,0.3,0.42));
#9675=CARTESIAN_POINT('',(40.,0.12,0.24));
#9676=CARTESIAN_POINT('Origin',(-0.1,-0.3,0.42));
#9677=CARTESIAN_POINT('',(0.,-0.3,0.42));
#9678=CARTESIAN_POINT('',(0.,-0.15,0.42));
#9679=CARTESIAN_POINT('',(40.,-0.3,0.42));
#9680=CARTESIAN_POINT('',(-0.1,-0.3,0.42));
#9681=CARTESIAN_POINT('',(40.,-0.15,0.42));
#9682=CARTESIAN_POINT('Origin',(-0.1,-0.55,0.67));
#9683=CARTESIAN_POINT('',(0.,-0.55,0.67));
#9684=CARTESIAN_POINT('',(6.93889390390723E-18,-0.245,0.365));
#9685=CARTESIAN_POINT('',(40.,-0.55,0.67));
#9686=CARTESIAN_POINT('',(-0.1,-0.55,0.67));
#9687=CARTESIAN_POINT('',(40.,-0.245,0.365));
#9688=CARTESIAN_POINT('Origin',(-0.1,-0.55,0.82));
#9689=CARTESIAN_POINT('',(0.,-0.55,0.82));
#9690=CARTESIAN_POINT('',(0.,-0.55,0.41));
#9691=CARTESIAN_POINT('',(40.,-0.55,0.82));
#9692=CARTESIAN_POINT('',(-0.1,-0.55,0.82));
#9693=CARTESIAN_POINT('',(40.,-0.55,0.41));
#9694=CARTESIAN_POINT('Origin',(-0.1,-0.3,0.82));
#9695=CARTESIAN_POINT('',(0.,-0.3,0.82));
#9696=CARTESIAN_POINT('',(0.,-0.15,0.82));
#9697=CARTESIAN_POINT('',(40.,-0.3,0.82));
#9698=CARTESIAN_POINT('',(-0.1,-0.3,0.82));
#9699=CARTESIAN_POINT('',(40.,-0.15,0.82));
#9700=CARTESIAN_POINT('Origin',(-0.1,-0.3,1.05));
#9701=CARTESIAN_POINT('',(0.,-0.3,1.));
#9702=CARTESIAN_POINT('',(0.,-0.3,0.525));
#9703=CARTESIAN_POINT('',(40.,-0.3,1.));
#9704=CARTESIAN_POINT('',(-0.05,-0.3,1.));
#9705=CARTESIAN_POINT('',(40.,-0.3,0.525));
#9706=CARTESIAN_POINT('Origin',(-0.1,0.,0.));
#9707=CARTESIAN_POINT('',(0.,-2.57175827820944E-17,0.21));
#9708=CARTESIAN_POINT('Origin',(0.,0.,0.));
#9709=CARTESIAN_POINT('',(40.,2.57175827820944E-17,0.21));
#9710=CARTESIAN_POINT('',(-0.1,-2.57175827820944E-17,0.21));
#9711=CARTESIAN_POINT('Origin',(40.,0.,0.));
#9712=CARTESIAN_POINT('Origin',(0.,1.,-1.));
#9713=CARTESIAN_POINT('',(0.,1.,1.));
#9714=CARTESIAN_POINT('',(0.,1.,-1.));
#9715=CARTESIAN_POINT('',(40.,1.,1.));
#9716=CARTESIAN_POINT('',(0.,1.,1.));
#9717=CARTESIAN_POINT('',(40.,1.,-1.));
#9718=CARTESIAN_POINT('Origin',(0.,1.,-1.));
#9719=CARTESIAN_POINT('',(40.,1.,-1.));
#9720=CARTESIAN_POINT('',(40.,1.,-1.));
#9721=CARTESIAN_POINT('',(0.,1.,-1.));
#9722=CARTESIAN_POINT('',(0.,1.,-1.));
#9723=CARTESIAN_POINT('',(0.,1.,-1.));
#9724=CARTESIAN_POINT('Origin',(0.,-1.,-1.));
#9725=CARTESIAN_POINT('',(0.,-1.,-1.));
#9726=CARTESIAN_POINT('',(40.,-1.,-1.));
#9727=CARTESIAN_POINT('Origin',(0.,-1.,-1.));
#9728=CARTESIAN_POINT('',(40.,-1.,-1.));
#9729=CARTESIAN_POINT('',(40.,-1.,-1.));
#9730=CARTESIAN_POINT('',(0.,-1.,-1.));
#9731=CARTESIAN_POINT('',(0.,-1.,-1.));
#9732=CARTESIAN_POINT('',(0.,-1.,-1.));
#9733=CARTESIAN_POINT('Origin',(0.,-1.,1.));
#9734=CARTESIAN_POINT('',(0.,-1.,1.));
#9735=CARTESIAN_POINT('',(40.,-1.,1.));
#9736=CARTESIAN_POINT('Origin',(0.,-1.,1.));
#9737=CARTESIAN_POINT('',(40.,-1.,1.));
#9738=CARTESIAN_POINT('',(40.,-1.,1.));
#9739=CARTESIAN_POINT('',(0.,-1.,1.));
#9740=CARTESIAN_POINT('',(0.,-1.,1.));
#9741=CARTESIAN_POINT('',(0.,-1.,1.));
#9742=CARTESIAN_POINT('Origin',(0.,1.,1.));
#9743=CARTESIAN_POINT('',(0.,1.,1.));
#9744=CARTESIAN_POINT('',(40.,1.,1.));
#9745=CARTESIAN_POINT('Origin',(0.,1.,1.));
#9746=CARTESIAN_POINT('',(40.,1.,1.));
#9747=CARTESIAN_POINT('',(0.,1.,1.));
#9748=CARTESIAN_POINT('Origin',(40.,0.,0.));
#9749=CARTESIAN_POINT('Origin',(0.,0.,0.));
#11653=UNCERTAINTY_MEASURE_WITH_UNIT(LENGTH_MEASURE(0.001),#11749,
'DISTANCE_ACCURACY_VALUE',
'Maximum model space distance between geometric entities at asserted c
onnectivities');
#11699=UNCERTAINTY_MEASURE_WITH_UNIT(LENGTH_MEASURE(0.001),#11749,
'DISTANCE_ACCURACY_VALUE',
'Maximum model space distance between geometric entities at asserted c
onnectivities');
#11702=(
GEOMETRIC_REPRESENTATION_CONTEXT(3)
GLOBAL_UNCERTAINTY_ASSIGNED_CONTEXT((#11653))
GLOBAL_UNIT_ASSIGNED_CONTEXT((#11749,#11751,#11752))
REPRESENTATION_CONTEXT('','3D')
);
#11748=(
GEOMETRIC_REPRESENTATION_CONTEXT(3)
GLOBAL_UNCERTAINTY_ASSIGNED_CONTEXT((#11699))
GLOBAL_UNIT_ASSIGNED_CONTEXT((#11749,#11751,#11752))
REPRESENTATION_CONTEXT('','3D')
);
#11749=(
LENGTH_UNIT()
NAMED_UNIT(*)
SI_UNIT(.CENTI.,.METRE.)
);
#11751=(
NAMED_UNIT(*)
PLANE_ANGLE_UNIT()
SI_UNIT($,.RADIAN.)
);
#11752=(
NAMED_UNIT(*)
SI_UNIT($,.STERADIAN.)
SOLID_ANGLE_UNIT()
);
#11755=SHAPE_DEFINITION_REPRESENTATION(#11803,#11926);
#11803=PRODUCT_DEFINITION_SHAPE('',$,#11975);
#11926=SHAPE_REPRESENTATION('',(#6736),#11702);
#11972=PRODUCT_DEFINITION_CONTEXT('part definition',#12118,'design');
#11975=PRODUCT_DEFINITION('Slotted Extrusion - 20 x 20 x 400 mm',
'Slotted Extrusion - 20 x 20 x 400 mm',#12023,#11972);
#12023=PRODUCT_DEFINITION_FORMATION('',$,#12122);
#12118=APPLICATION_CONTEXT(
'Core Data for Automotive Mechanical Design Process');
#12119=PRODUCT_CONTEXT('part definition',#12118,'mechanical');
#12122=PRODUCT('Slotted Extrusion - 20 x 20 x 400 mm',
'Slotted Extrusion - 20 x 20 x 400 mm',
'Slotted Extrusion - 20 x 20 x 400 mm',(#12119));
#12169=PRESENTATION_STYLE_ASSIGNMENT((#12174));
#12174=SURFACE_STYLE_USAGE(.BOTH.,#12179);
#12179=SURFACE_SIDE_STYLE('',(#12184));
#12184=SURFACE_STYLE_FILL_AREA(#12189);
#12189=FILL_AREA_STYLE('CAD Library Painted - Engineering blue',(#12194));
#12194=FILL_AREA_STYLE_COLOUR('CAD Library Painted - Engineering blue',
#12199);
#12199=COLOUR_RGB('CAD Library Painted - Engineering blue',0.12156862745098,
0.356862745098039,0.6);
ENDSEC;
END-ISO-10303-21;
